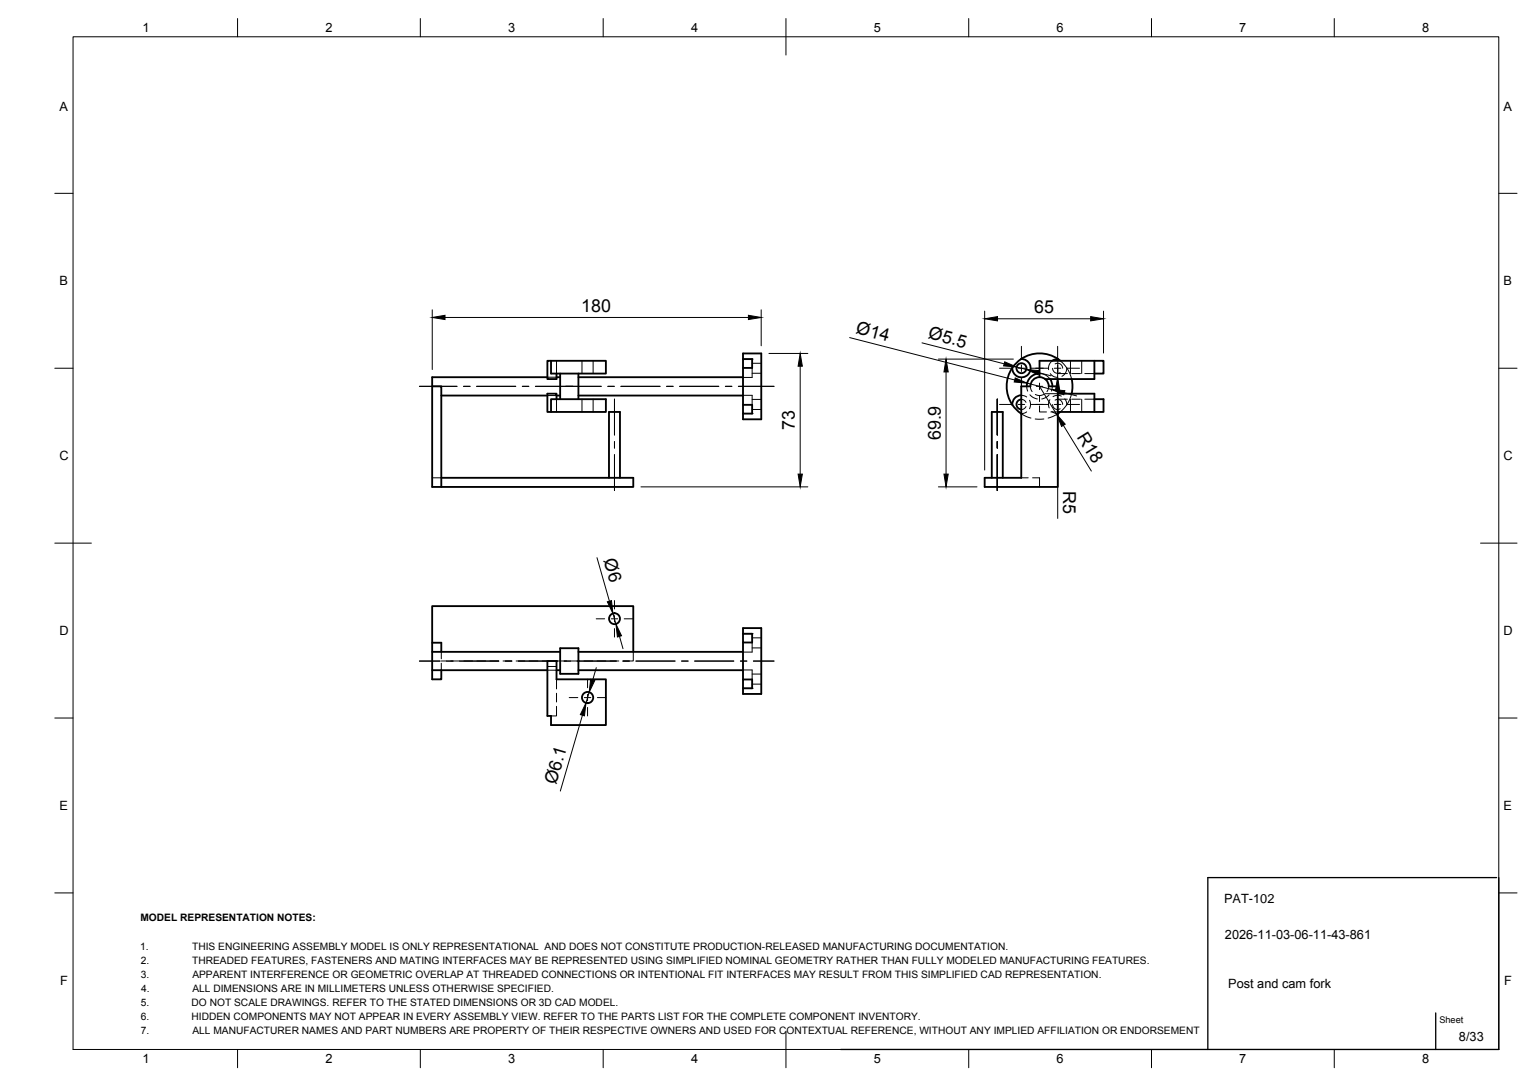
ISO-10303-21;
HEADER;
/* Generated by software containing ST-Developer
 * from STEP Tools, Inc. (www.steptools.com) 
 */

FILE_DESCRIPTION(
/* description */ ('Swing-away clamp arm'),
/* implementation_level */ '2;1');

FILE_NAME(
/* name */ 'Post and cam fork.step',
/* time_stamp */ '2026-10-28T03:26:03-07:00',
/* author */ (''),
/* organization */ (''),
/* preprocessor_version */ 'ST-DEVELOPER v20.2',
/* originating_system */ 'Autodesk Translation Framework v15.17.0.0',
/* authorisation */ '');

FILE_SCHEMA (('AUTOMOTIVE_DESIGN { 1 0 10303 214 3 1 1 }'));
ENDSEC;

DATA;
#10=MECHANICAL_DESIGN_GEOMETRIC_PRESENTATION_REPRESENTATION('',(#296),#10627);
#244=SHAPE_REPRESENTATION_RELATIONSHIP('SRR','None',#10742,#270);
#270=ADVANCED_BREP_SHAPE_REPRESENTATION('',(#330),#10601);
#296=STYLED_ITEM('',(#10958),#330);
#330=MANIFOLD_SOLID_BREP('Body1',#4902);
#366=FACE_BOUND('',#975,.T.);
#367=FACE_BOUND('',#978,.T.);
#368=FACE_BOUND('',#981,.T.);
#369=FACE_BOUND('',#984,.T.);
#370=FACE_BOUND('',#987,.T.);
#371=FACE_BOUND('',#992,.T.);
#372=FACE_BOUND('',#1004,.T.);
#373=FACE_BOUND('',#1005,.T.);
#374=FACE_BOUND('',#1012,.T.);
#375=FACE_BOUND('',#1018,.T.);
#376=FACE_BOUND('',#1022,.T.);
#377=FACE_BOUND('',#1028,.T.);
#378=FACE_BOUND('',#1039,.T.);
#379=FACE_BOUND('',#1042,.T.);
#380=FACE_BOUND('',#1045,.T.);
#381=FACE_BOUND('',#1046,.T.);
#382=FACE_BOUND('',#1047,.T.);
#383=FACE_BOUND('',#1048,.T.);
#476=PLANE('',#5259);
#477=PLANE('',#5265);
#478=PLANE('',#5271);
#479=PLANE('',#5277);
#480=PLANE('',#5283);
#481=PLANE('',#5295);
#482=PLANE('',#5296);
#483=PLANE('',#5297);
#484=PLANE('',#5298);
#485=PLANE('',#5299);
#486=PLANE('',#5300);
#487=PLANE('',#5301);
#488=PLANE('',#5303);
#489=PLANE('',#5304);
#490=PLANE('',#5305);
#491=PLANE('',#5306);
#492=PLANE('',#5307);
#493=PLANE('',#5318);
#494=PLANE('',#5319);
#495=PLANE('',#5320);
#496=PLANE('',#5321);
#497=PLANE('',#5322);
#498=PLANE('',#5323);
#499=PLANE('',#5324);
#500=PLANE('',#5325);
#501=PLANE('',#5326);
#502=PLANE('',#5327);
#503=PLANE('',#5328);
#504=PLANE('',#5332);
#505=PLANE('',#5333);
#506=PLANE('',#5334);
#507=PLANE('',#5335);
#508=PLANE('',#5336);
#509=PLANE('',#5337);
#510=PLANE('',#5338);
#511=PLANE('',#5339);
#512=PLANE('',#5340);
#513=PLANE('',#5341);
#514=PLANE('',#5342);
#515=PLANE('',#5351);
#516=PLANE('',#5356);
#517=PLANE('',#5358);
#659=FACE_OUTER_BOUND('',#974,.T.);
#660=FACE_OUTER_BOUND('',#976,.T.);
#661=FACE_OUTER_BOUND('',#977,.T.);
#662=FACE_OUTER_BOUND('',#979,.T.);
#663=FACE_OUTER_BOUND('',#980,.T.);
#664=FACE_OUTER_BOUND('',#982,.T.);
#665=FACE_OUTER_BOUND('',#983,.T.);
#666=FACE_OUTER_BOUND('',#985,.T.);
#667=FACE_OUTER_BOUND('',#986,.T.);
#668=FACE_OUTER_BOUND('',#988,.T.);
#669=FACE_OUTER_BOUND('',#989,.T.);
#670=FACE_OUTER_BOUND('',#990,.T.);
#671=FACE_OUTER_BOUND('',#991,.T.);
#672=FACE_OUTER_BOUND('',#993,.T.);
#673=FACE_OUTER_BOUND('',#994,.T.);
#674=FACE_OUTER_BOUND('',#995,.T.);
#675=FACE_OUTER_BOUND('',#996,.T.);
#676=FACE_OUTER_BOUND('',#997,.T.);
#677=FACE_OUTER_BOUND('',#998,.T.);
#678=FACE_OUTER_BOUND('',#999,.T.);
#679=FACE_OUTER_BOUND('',#1000,.T.);
#680=FACE_OUTER_BOUND('',#1001,.T.);
#681=FACE_OUTER_BOUND('',#1002,.T.);
#682=FACE_OUTER_BOUND('',#1003,.T.);
#683=FACE_OUTER_BOUND('',#1006,.T.);
#684=FACE_OUTER_BOUND('',#1007,.T.);
#685=FACE_OUTER_BOUND('',#1008,.T.);
#686=FACE_OUTER_BOUND('',#1009,.T.);
#687=FACE_OUTER_BOUND('',#1010,.T.);
#688=FACE_OUTER_BOUND('',#1011,.T.);
#689=FACE_OUTER_BOUND('',#1013,.T.);
#690=FACE_OUTER_BOUND('',#1014,.T.);
#691=FACE_OUTER_BOUND('',#1015,.T.);
#692=FACE_OUTER_BOUND('',#1016,.T.);
#693=FACE_OUTER_BOUND('',#1017,.T.);
#694=FACE_OUTER_BOUND('',#1019,.T.);
#695=FACE_OUTER_BOUND('',#1020,.T.);
#696=FACE_OUTER_BOUND('',#1021,.T.);
#697=FACE_OUTER_BOUND('',#1023,.T.);
#698=FACE_OUTER_BOUND('',#1024,.T.);
#699=FACE_OUTER_BOUND('',#1025,.T.);
#700=FACE_OUTER_BOUND('',#1026,.T.);
#701=FACE_OUTER_BOUND('',#1027,.T.);
#702=FACE_OUTER_BOUND('',#1029,.T.);
#703=FACE_OUTER_BOUND('',#1030,.T.);
#704=FACE_OUTER_BOUND('',#1031,.T.);
#705=FACE_OUTER_BOUND('',#1032,.T.);
#706=FACE_OUTER_BOUND('',#1033,.T.);
#707=FACE_OUTER_BOUND('',#1034,.T.);
#708=FACE_OUTER_BOUND('',#1035,.T.);
#709=FACE_OUTER_BOUND('',#1036,.T.);
#710=FACE_OUTER_BOUND('',#1037,.T.);
#711=FACE_OUTER_BOUND('',#1038,.T.);
#712=FACE_OUTER_BOUND('',#1040,.T.);
#713=FACE_OUTER_BOUND('',#1041,.T.);
#714=FACE_OUTER_BOUND('',#1043,.T.);
#715=FACE_OUTER_BOUND('',#1044,.T.);
#974=EDGE_LOOP('',(#3377,#3378));
#975=EDGE_LOOP('',(#3379));
#976=EDGE_LOOP('',(#3380,#3381,#3382,#3383));
#977=EDGE_LOOP('',(#3384,#3385));
#978=EDGE_LOOP('',(#3386));
#979=EDGE_LOOP('',(#3387,#3388,#3389,#3390));
#980=EDGE_LOOP('',(#3391,#3392));
#981=EDGE_LOOP('',(#3393));
#982=EDGE_LOOP('',(#3394,#3395,#3396,#3397));
#983=EDGE_LOOP('',(#3398,#3399));
#984=EDGE_LOOP('',(#3400));
#985=EDGE_LOOP('',(#3401,#3402,#3403,#3404));
#986=EDGE_LOOP('',(#3405,#3406,#3407,#3408,#3409,#3410,#3411,#3412,#3413));
#987=EDGE_LOOP('',(#3414));
#988=EDGE_LOOP('',(#3415,#3416,#3417,#3418,#3419,#3420,#3421,#3422,#3423,
#3424,#3425,#3426,#3427,#3428,#3429,#3430,#3431,#3432,#3433,#3434));
#989=EDGE_LOOP('',(#3435,#3436,#3437,#3438));
#990=EDGE_LOOP('',(#3439));
#991=EDGE_LOOP('',(#3440,#3441,#3442,#3443,#3444,#3445));
#992=EDGE_LOOP('',(#3446));
#993=EDGE_LOOP('',(#3447,#3448,#3449,#3450));
#994=EDGE_LOOP('',(#3451,#3452,#3453,#3454));
#995=EDGE_LOOP('',(#3455,#3456,#3457,#3458));
#996=EDGE_LOOP('',(#3459,#3460,#3461,#3462));
#997=EDGE_LOOP('',(#3463,#3464,#3465,#3466,#3467,#3468,#3469,#3470));
#998=EDGE_LOOP('',(#3471,#3472,#3473,#3474));
#999=EDGE_LOOP('',(#3475,#3476,#3477,#3478));
#1000=EDGE_LOOP('',(#3479,#3480,#3481,#3482));
#1001=EDGE_LOOP('',(#3483,#3484,#3485,#3486,#3487,#3488));
#1002=EDGE_LOOP('',(#3489,#3490,#3491,#3492,#3493,#3494,#3495,#3496));
#1003=EDGE_LOOP('',(#3497,#3498,#3499,#3500,#3501,#3502,#3503));
#1004=EDGE_LOOP('',(#3504,#3505,#3506,#3507));
#1005=EDGE_LOOP('',(#3508,#3509,#3510,#3511));
#1006=EDGE_LOOP('',(#3512,#3513,#3514,#3515));
#1007=EDGE_LOOP('',(#3516,#3517,#3518,#3519));
#1008=EDGE_LOOP('',(#3520,#3521,#3522,#3523));
#1009=EDGE_LOOP('',(#3524,#3525,#3526,#3527));
#1010=EDGE_LOOP('',(#3528,#3529,#3530,#3531));
#1011=EDGE_LOOP('',(#3532,#3533,#3534,#3535,#3536,#3537));
#1012=EDGE_LOOP('',(#3538));
#1013=EDGE_LOOP('',(#3539,#3540,#3541,#3542,#3543,#3544,#3545));
#1014=EDGE_LOOP('',(#3546,#3547,#3548,#3549,#3550,#3551));
#1015=EDGE_LOOP('',(#3552,#3553,#3554,#3555));
#1016=EDGE_LOOP('',(#3556,#3557,#3558,#3559,#3560));
#1017=EDGE_LOOP('',(#3561,#3562,#3563,#3564,#3565,#3566,#3567,#3568));
#1018=EDGE_LOOP('',(#3569));
#1019=EDGE_LOOP('',(#3570,#3571,#3572,#3573));
#1020=EDGE_LOOP('',(#3574,#3575,#3576,#3577));
#1021=EDGE_LOOP('',(#3578,#3579,#3580,#3581,#3582,#3583));
#1022=EDGE_LOOP('',(#3584));
#1023=EDGE_LOOP('',(#3585,#3586,#3587,#3588));
#1024=EDGE_LOOP('',(#3589,#3590,#3591,#3592));
#1025=EDGE_LOOP('',(#3593,#3594,#3595,#3596));
#1026=EDGE_LOOP('',(#3597,#3598,#3599,#3600));
#1027=EDGE_LOOP('',(#3601,#3602,#3603,#3604,#3605,#3606,#3607,#3608));
#1028=EDGE_LOOP('',(#3609));
#1029=EDGE_LOOP('',(#3610,#3611,#3612,#3613,#3614));
#1030=EDGE_LOOP('',(#3615,#3616,#3617,#3618));
#1031=EDGE_LOOP('',(#3619,#3620,#3621,#3622,#3623,#3624,#3625));
#1032=EDGE_LOOP('',(#3626,#3627,#3628,#3629,#3630,#3631));
#1033=EDGE_LOOP('',(#3632,#3633,#3634,#3635));
#1034=EDGE_LOOP('',(#3636,#3637,#3638,#3639));
#1035=EDGE_LOOP('',(#3640,#3641,#3642,#3643));
#1036=EDGE_LOOP('',(#3644,#3645,#3646,#3647));
#1037=EDGE_LOOP('',(#3648,#3649,#3650,#3651));
#1038=EDGE_LOOP('',(#3652));
#1039=EDGE_LOOP('',(#3653));
#1040=EDGE_LOOP('',(#3654,#3655,#3656,#3657));
#1041=EDGE_LOOP('',(#3658));
#1042=EDGE_LOOP('',(#3659));
#1043=EDGE_LOOP('',(#3660,#3661,#3662,#3663));
#1044=EDGE_LOOP('',(#3664));
#1045=EDGE_LOOP('',(#3665));
#1046=EDGE_LOOP('',(#3666));
#1047=EDGE_LOOP('',(#3667));
#1048=EDGE_LOOP('',(#3668));
#1391=LINE('',#7603,#1713);
#1392=LINE('',#7606,#1714);
#1393=LINE('',#7616,#1715);
#1394=LINE('',#7619,#1716);
#1395=LINE('',#7629,#1717);
#1396=LINE('',#7632,#1718);
#1397=LINE('',#7642,#1719);
#1398=LINE('',#7645,#1720);
#1399=LINE('',#7657,#1721);
#1400=LINE('',#7663,#1722);
#1401=LINE('',#7669,#1723);
#1402=LINE('',#7671,#1724);
#1403=LINE('',#7673,#1725);
#1404=LINE('',#7675,#1726);
#1405=LINE('',#7677,#1727);
#1406=LINE('',#7678,#1728);
#1407=LINE('',#7681,#1729);
#1408=LINE('',#7683,#1730);
#1409=LINE('',#7684,#1731);
#1410=LINE('',#7688,#1732);
#1411=LINE('',#7689,#1733);
#1412=LINE('',#7690,#1734);
#1413=LINE('',#7692,#1735);
#1414=LINE('',#7695,#1736);
#1415=LINE('',#7697,#1737);
#1416=LINE('',#7698,#1738);
#1417=LINE('',#7701,#1739);
#1418=LINE('',#7703,#1740);
#1419=LINE('',#7705,#1741);
#1420=LINE('',#7708,#1742);
#1421=LINE('',#7711,#1743);
#1422=LINE('',#7712,#1744);
#1423=LINE('',#7715,#1745);
#1424=LINE('',#7717,#1746);
#1425=LINE('',#7718,#1747);
#1426=LINE('',#7721,#1748);
#1427=LINE('',#7722,#1749);
#1428=LINE('',#7724,#1750);
#1429=LINE('',#7729,#1751);
#1430=LINE('',#7733,#1752);
#1431=LINE('',#7737,#1753);
#1432=LINE('',#7741,#1754);
#1433=LINE('',#7745,#1755);
#1434=LINE('',#7751,#1756);
#1435=LINE('',#7756,#1757);
#1436=LINE('',#7758,#1758);
#1437=LINE('',#7760,#1759);
#1438=LINE('',#7761,#1760);
#1439=LINE('',#7765,#1761);
#1440=LINE('',#7767,#1762);
#1441=LINE('',#7769,#1763);
#1442=LINE('',#7770,#1764);
#1443=LINE('',#7773,#1765);
#1444=LINE('',#7775,#1766);
#1445=LINE('',#7776,#1767);
#1446=LINE('',#7778,#1768);
#1447=LINE('',#7779,#1769);
#1448=LINE('',#7782,#1770);
#1449=LINE('',#7783,#1771);
#1450=LINE('',#7786,#1772);
#1451=LINE('',#7787,#1773);
#1452=LINE('',#7789,#1774);
#1453=LINE('',#7790,#1775);
#1454=LINE('',#7793,#1776);
#1455=LINE('',#7795,#1777);
#1456=LINE('',#7796,#1778);
#1457=LINE('',#7799,#1779);
#1458=LINE('',#7800,#1780);
#1459=LINE('',#7802,#1781);
#1460=LINE('',#7803,#1782);
#1461=LINE('',#7810,#1783);
#1462=LINE('',#7815,#1784);
#1463=LINE('',#7817,#1785);
#1464=LINE('',#7819,#1786);
#1465=LINE('',#7821,#1787);
#1466=LINE('',#7823,#1788);
#1467=LINE('',#7824,#1789);
#1468=LINE('',#7827,#1790);
#1469=LINE('',#7829,#1791);
#1470=LINE('',#7830,#1792);
#1471=LINE('',#7833,#1793);
#1472=LINE('',#7835,#1794);
#1473=LINE('',#7836,#1795);
#1474=LINE('',#7839,#1796);
#1475=LINE('',#7840,#1797);
#1476=LINE('',#7842,#1798);
#1477=LINE('',#7845,#1799);
#1478=LINE('',#7847,#1800);
#1479=LINE('',#7849,#1801);
#1480=LINE('',#7850,#1802);
#1481=LINE('',#7852,#1803);
#1482=LINE('',#7854,#1804);
#1483=LINE('',#7855,#1805);
#1484=LINE('',#7857,#1806);
#1485=LINE('',#7860,#1807);
#1486=LINE('',#7861,#1808);
#1487=LINE('',#7863,#1809);
#1488=LINE('',#7868,#1810);
#1489=LINE('',#7872,#1811);
#1490=LINE('',#7876,#1812);
#1491=LINE('',#7880,#1813);
#1492=LINE('',#7889,#1814);
#1493=LINE('',#7892,#1815);
#1713=VECTOR('',#5992,1.);
#1714=VECTOR('',#5995,1.);
#1715=VECTOR('',#6006,1.);
#1716=VECTOR('',#6009,1.);
#1717=VECTOR('',#6020,1.);
#1718=VECTOR('',#6023,1.);
#1719=VECTOR('',#6034,1.);
#1720=VECTOR('',#6037,1.);
#1721=VECTOR('',#6054,1.8);
#1722=VECTOR('',#6061,0.3);
#1723=VECTOR('',#6068,1.);
#1724=VECTOR('',#6069,1.);
#1725=VECTOR('',#6070,1.);
#1726=VECTOR('',#6071,1.);
#1727=VECTOR('',#6072,1.);
#1728=VECTOR('',#6073,1.);
#1729=VECTOR('',#6076,1.);
#1730=VECTOR('',#6077,1.);
#1731=VECTOR('',#6078,1.);
#1732=VECTOR('',#6081,1.);
#1733=VECTOR('',#6082,1.);
#1734=VECTOR('',#6083,1.);
#1735=VECTOR('',#6086,1.);
#1736=VECTOR('',#6089,1.);
#1737=VECTOR('',#6090,1.);
#1738=VECTOR('',#6091,1.);
#1739=VECTOR('',#6094,1.);
#1740=VECTOR('',#6095,1.);
#1741=VECTOR('',#6096,1.);
#1742=VECTOR('',#6099,1.);
#1743=VECTOR('',#6102,1.);
#1744=VECTOR('',#6103,1.);
#1745=VECTOR('',#6106,1.);
#1746=VECTOR('',#6107,1.);
#1747=VECTOR('',#6108,1.);
#1748=VECTOR('',#6111,1.);
#1749=VECTOR('',#6112,1.);
#1750=VECTOR('',#6115,1.);
#1751=VECTOR('',#6122,0.5);
#1752=VECTOR('',#6125,1.);
#1753=VECTOR('',#6128,1.);
#1754=VECTOR('',#6131,1.);
#1755=VECTOR('',#6134,1.);
#1756=VECTOR('',#6141,0.305);
#1757=VECTOR('',#6146,1.);
#1758=VECTOR('',#6147,1.);
#1759=VECTOR('',#6148,1.);
#1760=VECTOR('',#6149,1.);
#1761=VECTOR('',#6152,1.);
#1762=VECTOR('',#6153,1.);
#1763=VECTOR('',#6154,1.);
#1764=VECTOR('',#6155,1.);
#1765=VECTOR('',#6158,1.);
#1766=VECTOR('',#6159,1.);
#1767=VECTOR('',#6160,1.);
#1768=VECTOR('',#6163,1.);
#1769=VECTOR('',#6164,1.);
#1770=VECTOR('',#6167,1.);
#1771=VECTOR('',#6168,1.);
#1772=VECTOR('',#6171,1.);
#1773=VECTOR('',#6172,1.);
#1774=VECTOR('',#6173,1.);
#1775=VECTOR('',#6174,1.);
#1776=VECTOR('',#6177,1.);
#1777=VECTOR('',#6178,1.);
#1778=VECTOR('',#6179,1.);
#1779=VECTOR('',#6182,1.);
#1780=VECTOR('',#6183,1.);
#1781=VECTOR('',#6186,1.);
#1782=VECTOR('',#6187,1.);
#1783=VECTOR('',#6196,0.305);
#1784=VECTOR('',#6201,1.);
#1785=VECTOR('',#6202,1.);
#1786=VECTOR('',#6203,1.);
#1787=VECTOR('',#6204,1.);
#1788=VECTOR('',#6205,1.);
#1789=VECTOR('',#6206,1.);
#1790=VECTOR('',#6209,1.);
#1791=VECTOR('',#6210,1.);
#1792=VECTOR('',#6211,1.);
#1793=VECTOR('',#6214,1.);
#1794=VECTOR('',#6215,1.);
#1795=VECTOR('',#6216,1.);
#1796=VECTOR('',#6219,1.);
#1797=VECTOR('',#6220,1.);
#1798=VECTOR('',#6223,1.);
#1799=VECTOR('',#6226,1.);
#1800=VECTOR('',#6227,1.);
#1801=VECTOR('',#6228,1.);
#1802=VECTOR('',#6229,1.);
#1803=VECTOR('',#6232,1.);
#1804=VECTOR('',#6233,1.);
#1805=VECTOR('',#6234,1.);
#1806=VECTOR('',#6237,1.);
#1807=VECTOR('',#6240,1.);
#1808=VECTOR('',#6241,1.);
#1809=VECTOR('',#6244,1.);
#1810=VECTOR('',#6251,0.275);
#1811=VECTOR('',#6256,0.275);
#1812=VECTOR('',#6261,0.275);
#1813=VECTOR('',#6266,0.275);
#1814=VECTOR('',#6277,0.7);
#1815=VECTOR('',#6282,0.5);
#2003=CIRCLE('',#5260,1.8);
#2004=CIRCLE('',#5261,0.5);
#2005=CIRCLE('',#5262,0.275);
#2006=CIRCLE('',#5264,0.5);
#2007=CIRCLE('',#5266,1.8);
#2008=CIRCLE('',#5267,0.5);
#2009=CIRCLE('',#5268,0.275);
#2010=CIRCLE('',#5270,0.5);
#2011=CIRCLE('',#5272,1.8);
#2012=CIRCLE('',#5273,0.5);
#2013=CIRCLE('',#5274,0.275);
#2014=CIRCLE('',#5276,0.5);
#2015=CIRCLE('',#5278,1.8);
#2016=CIRCLE('',#5279,0.5);
#2017=CIRCLE('',#5280,0.275);
#2018=CIRCLE('',#5282,0.5);
#2019=CIRCLE('',#5284,1.8);
#2020=CIRCLE('',#5285,1.8);
#2021=CIRCLE('',#5286,1.8);
#2022=CIRCLE('',#5287,1.8);
#2023=CIRCLE('',#5288,1.8);
#2024=CIRCLE('',#5289,0.5);
#2025=CIRCLE('',#5291,1.8);
#2026=CIRCLE('',#5293,0.3);
#2027=CIRCLE('',#5294,0.3);
#2028=CIRCLE('',#5302,0.5);
#2029=CIRCLE('',#5308,0.5);
#2030=CIRCLE('',#5310,0.5);
#2031=CIRCLE('',#5311,0.5);
#2032=CIRCLE('',#5312,0.5);
#2033=CIRCLE('',#5313,0.5);
#2034=CIRCLE('',#5314,0.5);
#2035=CIRCLE('',#5316,0.305);
#2036=CIRCLE('',#5317,0.305);
#2037=CIRCLE('',#5330,0.305);
#2038=CIRCLE('',#5331,0.305);
#2039=CIRCLE('',#5344,0.275);
#2040=CIRCLE('',#5346,0.275);
#2041=CIRCLE('',#5348,0.275);
#2042=CIRCLE('',#5350,0.275);
#2043=CIRCLE('',#5352,0.7);
#2044=CIRCLE('',#5353,0.5);
#2045=CIRCLE('',#5355,0.7);
#2294=VERTEX_POINT('',#7595);
#2295=VERTEX_POINT('',#7596);
#2296=VERTEX_POINT('',#7599);
#2297=VERTEX_POINT('',#7602);
#2298=VERTEX_POINT('',#7604);
#2299=VERTEX_POINT('',#7608);
#2300=VERTEX_POINT('',#7609);
#2301=VERTEX_POINT('',#7612);
#2302=VERTEX_POINT('',#7615);
#2303=VERTEX_POINT('',#7617);
#2304=VERTEX_POINT('',#7621);
#2305=VERTEX_POINT('',#7622);
#2306=VERTEX_POINT('',#7625);
#2307=VERTEX_POINT('',#7628);
#2308=VERTEX_POINT('',#7630);
#2309=VERTEX_POINT('',#7634);
#2310=VERTEX_POINT('',#7635);
#2311=VERTEX_POINT('',#7638);
#2312=VERTEX_POINT('',#7641);
#2313=VERTEX_POINT('',#7643);
#2314=VERTEX_POINT('',#7650);
#2315=VERTEX_POINT('',#7653);
#2316=VERTEX_POINT('',#7656);
#2317=VERTEX_POINT('',#7660);
#2318=VERTEX_POINT('',#7662);
#2319=VERTEX_POINT('',#7667);
#2320=VERTEX_POINT('',#7668);
#2321=VERTEX_POINT('',#7670);
#2322=VERTEX_POINT('',#7672);
#2323=VERTEX_POINT('',#7674);
#2324=VERTEX_POINT('',#7676);
#2325=VERTEX_POINT('',#7680);
#2326=VERTEX_POINT('',#7682);
#2327=VERTEX_POINT('',#7686);
#2328=VERTEX_POINT('',#7687);
#2329=VERTEX_POINT('',#7694);
#2330=VERTEX_POINT('',#7696);
#2331=VERTEX_POINT('',#7700);
#2332=VERTEX_POINT('',#7702);
#2333=VERTEX_POINT('',#7704);
#2334=VERTEX_POINT('',#7706);
#2335=VERTEX_POINT('',#7710);
#2336=VERTEX_POINT('',#7714);
#2337=VERTEX_POINT('',#7716);
#2338=VERTEX_POINT('',#7720);
#2339=VERTEX_POINT('',#7728);
#2340=VERTEX_POINT('',#7731);
#2341=VERTEX_POINT('',#7732);
#2342=VERTEX_POINT('',#7734);
#2343=VERTEX_POINT('',#7736);
#2344=VERTEX_POINT('',#7739);
#2345=VERTEX_POINT('',#7740);
#2346=VERTEX_POINT('',#7742);
#2347=VERTEX_POINT('',#7744);
#2348=VERTEX_POINT('',#7748);
#2349=VERTEX_POINT('',#7750);
#2350=VERTEX_POINT('',#7754);
#2351=VERTEX_POINT('',#7755);
#2352=VERTEX_POINT('',#7757);
#2353=VERTEX_POINT('',#7759);
#2354=VERTEX_POINT('',#7763);
#2355=VERTEX_POINT('',#7764);
#2356=VERTEX_POINT('',#7766);
#2357=VERTEX_POINT('',#7768);
#2358=VERTEX_POINT('',#7772);
#2359=VERTEX_POINT('',#7774);
#2360=VERTEX_POINT('',#7781);
#2361=VERTEX_POINT('',#7785);
#2362=VERTEX_POINT('',#7788);
#2363=VERTEX_POINT('',#7792);
#2364=VERTEX_POINT('',#7794);
#2365=VERTEX_POINT('',#7798);
#2366=VERTEX_POINT('',#7807);
#2367=VERTEX_POINT('',#7809);
#2368=VERTEX_POINT('',#7813);
#2369=VERTEX_POINT('',#7814);
#2370=VERTEX_POINT('',#7816);
#2371=VERTEX_POINT('',#7818);
#2372=VERTEX_POINT('',#7820);
#2373=VERTEX_POINT('',#7822);
#2374=VERTEX_POINT('',#7826);
#2375=VERTEX_POINT('',#7828);
#2376=VERTEX_POINT('',#7832);
#2377=VERTEX_POINT('',#7834);
#2378=VERTEX_POINT('',#7838);
#2379=VERTEX_POINT('',#7844);
#2380=VERTEX_POINT('',#7846);
#2381=VERTEX_POINT('',#7848);
#2382=VERTEX_POINT('',#7853);
#2383=VERTEX_POINT('',#7859);
#2384=VERTEX_POINT('',#7866);
#2385=VERTEX_POINT('',#7870);
#2386=VERTEX_POINT('',#7874);
#2387=VERTEX_POINT('',#7878);
#2388=VERTEX_POINT('',#7882);
#2389=VERTEX_POINT('',#7884);
#2390=VERTEX_POINT('',#7887);
#2721=EDGE_CURVE('',#2294,#2295,#2003,.T.);
#2722=EDGE_CURVE('',#2294,#2295,#2004,.T.);
#2723=EDGE_CURVE('',#2296,#2296,#2005,.T.);
#2724=EDGE_CURVE('',#2297,#2294,#1391,.T.);
#2725=EDGE_CURVE('',#2298,#2297,#2006,.T.);
#2726=EDGE_CURVE('',#2295,#2298,#1392,.T.);
#2727=EDGE_CURVE('',#2299,#2300,#2007,.T.);
#2728=EDGE_CURVE('',#2299,#2300,#2008,.T.);
#2729=EDGE_CURVE('',#2301,#2301,#2009,.T.);
#2730=EDGE_CURVE('',#2302,#2299,#1393,.T.);
#2731=EDGE_CURVE('',#2303,#2302,#2010,.T.);
#2732=EDGE_CURVE('',#2300,#2303,#1394,.T.);
#2733=EDGE_CURVE('',#2304,#2305,#2011,.T.);
#2734=EDGE_CURVE('',#2304,#2305,#2012,.T.);
#2735=EDGE_CURVE('',#2306,#2306,#2013,.T.);
#2736=EDGE_CURVE('',#2307,#2304,#1395,.T.);
#2737=EDGE_CURVE('',#2308,#2307,#2014,.T.);
#2738=EDGE_CURVE('',#2305,#2308,#1396,.T.);
#2739=EDGE_CURVE('',#2309,#2310,#2015,.T.);
#2740=EDGE_CURVE('',#2309,#2310,#2016,.T.);
#2741=EDGE_CURVE('',#2311,#2311,#2017,.T.);
#2742=EDGE_CURVE('',#2312,#2309,#1397,.T.);
#2743=EDGE_CURVE('',#2313,#2312,#2018,.T.);
#2744=EDGE_CURVE('',#2310,#2313,#1398,.T.);
#2745=EDGE_CURVE('',#2297,#2313,#2019,.T.);
#2746=EDGE_CURVE('',#2312,#2308,#2020,.T.);
#2747=EDGE_CURVE('',#2307,#2303,#2021,.T.);
#2748=EDGE_CURVE('',#2302,#2314,#2022,.T.);
#2749=EDGE_CURVE('',#2314,#2298,#2023,.T.);
#2750=EDGE_CURVE('',#2315,#2315,#2024,.T.);
#2751=EDGE_CURVE('',#2314,#2316,#1399,.T.);
#2752=EDGE_CURVE('',#2316,#2316,#2025,.T.);
#2753=EDGE_CURVE('',#2317,#2317,#2026,.T.);
#2754=EDGE_CURVE('',#2317,#2318,#1400,.T.);
#2755=EDGE_CURVE('',#2318,#2318,#2027,.T.);
#2756=EDGE_CURVE('',#2319,#2320,#1401,.T.);
#2757=EDGE_CURVE('',#2321,#2319,#1402,.T.);
#2758=EDGE_CURVE('',#2321,#2322,#1403,.T.);
#2759=EDGE_CURVE('',#2322,#2323,#1404,.T.);
#2760=EDGE_CURVE('',#2323,#2324,#1405,.T.);
#2761=EDGE_CURVE('',#2324,#2320,#1406,.T.);
#2762=EDGE_CURVE('',#2325,#2321,#1407,.T.);
#2763=EDGE_CURVE('',#2326,#2325,#1408,.T.);
#2764=EDGE_CURVE('',#2326,#2322,#1409,.T.);
#2765=EDGE_CURVE('',#2327,#2328,#1410,.T.);
#2766=EDGE_CURVE('',#2327,#2324,#1411,.T.);
#2767=EDGE_CURVE('',#2328,#2323,#1412,.T.);
#2768=EDGE_CURVE('',#2328,#2326,#1413,.T.);
#2769=EDGE_CURVE('',#2329,#2320,#1414,.T.);
#2770=EDGE_CURVE('',#2330,#2329,#1415,.T.);
#2771=EDGE_CURVE('',#2330,#2319,#1416,.T.);
#2772=EDGE_CURVE('',#2331,#2327,#1417,.T.);
#2773=EDGE_CURVE('',#2331,#2332,#1418,.T.);
#2774=EDGE_CURVE('',#2332,#2333,#1419,.T.);
#2775=EDGE_CURVE('',#2333,#2334,#2028,.T.);
#2776=EDGE_CURVE('',#2334,#2329,#1420,.T.);
#2777=EDGE_CURVE('',#2335,#2334,#1421,.T.);
#2778=EDGE_CURVE('',#2335,#2330,#1422,.T.);
#2779=EDGE_CURVE('',#2333,#2336,#1423,.T.);
#2780=EDGE_CURVE('',#2337,#2332,#1424,.T.);
#2781=EDGE_CURVE('',#2337,#2336,#1425,.T.);
#2782=EDGE_CURVE('',#2338,#2337,#1426,.T.);
#2783=EDGE_CURVE('',#2338,#2331,#1427,.T.);
#2784=EDGE_CURVE('',#2325,#2338,#1428,.T.);
#2785=EDGE_CURVE('',#2336,#2335,#2029,.T.);
#2786=EDGE_CURVE('',#2335,#2339,#1429,.T.);
#2787=EDGE_CURVE('',#2339,#2339,#2030,.T.);
#2788=EDGE_CURVE('',#2340,#2341,#1430,.T.);
#2789=EDGE_CURVE('',#2341,#2342,#2031,.T.);
#2790=EDGE_CURVE('',#2342,#2343,#1431,.T.);
#2791=EDGE_CURVE('',#2343,#2340,#2032,.T.);
#2792=EDGE_CURVE('',#2344,#2345,#1432,.T.);
#2793=EDGE_CURVE('',#2345,#2346,#2033,.T.);
#2794=EDGE_CURVE('',#2346,#2347,#1433,.T.);
#2795=EDGE_CURVE('',#2347,#2344,#2034,.T.);
#2796=EDGE_CURVE('',#2348,#2348,#2035,.T.);
#2797=EDGE_CURVE('',#2348,#2349,#1434,.T.);
#2798=EDGE_CURVE('',#2349,#2349,#2036,.T.);
#2799=EDGE_CURVE('',#2350,#2351,#1435,.T.);
#2800=EDGE_CURVE('',#2352,#2350,#1436,.T.);
#2801=EDGE_CURVE('',#2352,#2353,#1437,.T.);
#2802=EDGE_CURVE('',#2351,#2353,#1438,.T.);
#2803=EDGE_CURVE('',#2354,#2355,#1439,.T.);
#2804=EDGE_CURVE('',#2356,#2354,#1440,.T.);
#2805=EDGE_CURVE('',#2357,#2356,#1441,.T.);
#2806=EDGE_CURVE('',#2355,#2357,#1442,.T.);
#2807=EDGE_CURVE('',#2357,#2358,#1443,.T.);
#2808=EDGE_CURVE('',#2359,#2356,#1444,.T.);
#2809=EDGE_CURVE('',#2358,#2359,#1445,.T.);
#2810=EDGE_CURVE('',#2358,#2352,#1446,.T.);
#2811=EDGE_CURVE('',#2353,#2359,#1447,.T.);
#2812=EDGE_CURVE('',#2355,#2360,#1448,.T.);
#2813=EDGE_CURVE('',#2360,#2350,#1449,.T.);
#2814=EDGE_CURVE('',#2361,#2360,#1450,.T.);
#2815=EDGE_CURVE('',#2346,#2361,#1451,.T.);
#2816=EDGE_CURVE('',#2345,#2362,#1452,.T.);
#2817=EDGE_CURVE('',#2354,#2362,#1453,.T.);
#2818=EDGE_CURVE('',#2363,#2351,#1454,.T.);
#2819=EDGE_CURVE('',#2364,#2363,#1455,.T.);
#2820=EDGE_CURVE('',#2361,#2364,#1456,.T.);
#2821=EDGE_CURVE('',#2344,#2365,#1457,.T.);
#2822=EDGE_CURVE('',#2362,#2365,#1458,.T.);
#2823=EDGE_CURVE('',#2364,#2347,#1459,.T.);
#2824=EDGE_CURVE('',#2365,#2363,#1460,.T.);
#2825=EDGE_CURVE('',#2366,#2366,#2037,.T.);
#2826=EDGE_CURVE('',#2366,#2367,#1461,.T.);
#2827=EDGE_CURVE('',#2367,#2367,#2038,.T.);
#2828=EDGE_CURVE('',#2368,#2369,#1462,.T.);
#2829=EDGE_CURVE('',#2370,#2368,#1463,.T.);
#2830=EDGE_CURVE('',#2370,#2371,#1464,.T.);
#2831=EDGE_CURVE('',#2371,#2372,#1465,.T.);
#2832=EDGE_CURVE('',#2372,#2373,#1466,.T.);
#2833=EDGE_CURVE('',#2373,#2369,#1467,.T.);
#2834=EDGE_CURVE('',#2374,#2370,#1468,.T.);
#2835=EDGE_CURVE('',#2375,#2374,#1469,.T.);
#2836=EDGE_CURVE('',#2375,#2371,#1470,.T.);
#2837=EDGE_CURVE('',#2369,#2376,#1471,.T.);
#2838=EDGE_CURVE('',#2377,#2373,#1472,.T.);
#2839=EDGE_CURVE('',#2376,#2377,#1473,.T.);
#2840=EDGE_CURVE('',#2377,#2378,#1474,.T.);
#2841=EDGE_CURVE('',#2378,#2372,#1475,.T.);
#2842=EDGE_CURVE('',#2378,#2375,#1476,.T.);
#2843=EDGE_CURVE('',#2374,#2379,#1477,.T.);
#2844=EDGE_CURVE('',#2379,#2380,#1478,.T.);
#2845=EDGE_CURVE('',#2380,#2381,#1479,.T.);
#2846=EDGE_CURVE('',#2381,#2376,#1480,.T.);
#2847=EDGE_CURVE('',#2380,#2341,#1481,.T.);
#2848=EDGE_CURVE('',#2379,#2382,#1482,.T.);
#2849=EDGE_CURVE('',#2342,#2382,#1483,.T.);
#2850=EDGE_CURVE('',#2381,#2340,#1484,.T.);
#2851=EDGE_CURVE('',#2383,#2343,#1485,.T.);
#2852=EDGE_CURVE('',#2368,#2383,#1486,.T.);
#2853=EDGE_CURVE('',#2382,#2383,#1487,.T.);
#2854=EDGE_CURVE('',#2384,#2384,#2039,.T.);
#2855=EDGE_CURVE('',#2384,#2296,#1488,.T.);
#2856=EDGE_CURVE('',#2385,#2385,#2040,.T.);
#2857=EDGE_CURVE('',#2385,#2301,#1489,.T.);
#2858=EDGE_CURVE('',#2386,#2386,#2041,.T.);
#2859=EDGE_CURVE('',#2386,#2306,#1490,.T.);
#2860=EDGE_CURVE('',#2387,#2387,#2042,.T.);
#2861=EDGE_CURVE('',#2387,#2311,#1491,.T.);
#2862=EDGE_CURVE('',#2388,#2388,#2043,.T.);
#2863=EDGE_CURVE('',#2389,#2389,#2044,.T.);
#2864=EDGE_CURVE('',#2390,#2390,#2045,.T.);
#2865=EDGE_CURVE('',#2390,#2388,#1492,.T.);
#2866=EDGE_CURVE('',#2389,#2315,#1493,.T.);
#3377=ORIENTED_EDGE('',*,*,#2721,.F.);
#3378=ORIENTED_EDGE('',*,*,#2722,.T.);
#3379=ORIENTED_EDGE('',*,*,#2723,.F.);
#3380=ORIENTED_EDGE('',*,*,#2724,.F.);
#3381=ORIENTED_EDGE('',*,*,#2725,.F.);
#3382=ORIENTED_EDGE('',*,*,#2726,.F.);
#3383=ORIENTED_EDGE('',*,*,#2722,.F.);
#3384=ORIENTED_EDGE('',*,*,#2727,.F.);
#3385=ORIENTED_EDGE('',*,*,#2728,.T.);
#3386=ORIENTED_EDGE('',*,*,#2729,.F.);
#3387=ORIENTED_EDGE('',*,*,#2730,.F.);
#3388=ORIENTED_EDGE('',*,*,#2731,.F.);
#3389=ORIENTED_EDGE('',*,*,#2732,.F.);
#3390=ORIENTED_EDGE('',*,*,#2728,.F.);
#3391=ORIENTED_EDGE('',*,*,#2733,.F.);
#3392=ORIENTED_EDGE('',*,*,#2734,.T.);
#3393=ORIENTED_EDGE('',*,*,#2735,.F.);
#3394=ORIENTED_EDGE('',*,*,#2736,.F.);
#3395=ORIENTED_EDGE('',*,*,#2737,.F.);
#3396=ORIENTED_EDGE('',*,*,#2738,.F.);
#3397=ORIENTED_EDGE('',*,*,#2734,.F.);
#3398=ORIENTED_EDGE('',*,*,#2739,.F.);
#3399=ORIENTED_EDGE('',*,*,#2740,.T.);
#3400=ORIENTED_EDGE('',*,*,#2741,.F.);
#3401=ORIENTED_EDGE('',*,*,#2742,.F.);
#3402=ORIENTED_EDGE('',*,*,#2743,.F.);
#3403=ORIENTED_EDGE('',*,*,#2744,.F.);
#3404=ORIENTED_EDGE('',*,*,#2740,.F.);
#3405=ORIENTED_EDGE('',*,*,#2725,.T.);
#3406=ORIENTED_EDGE('',*,*,#2745,.T.);
#3407=ORIENTED_EDGE('',*,*,#2743,.T.);
#3408=ORIENTED_EDGE('',*,*,#2746,.T.);
#3409=ORIENTED_EDGE('',*,*,#2737,.T.);
#3410=ORIENTED_EDGE('',*,*,#2747,.T.);
#3411=ORIENTED_EDGE('',*,*,#2731,.T.);
#3412=ORIENTED_EDGE('',*,*,#2748,.T.);
#3413=ORIENTED_EDGE('',*,*,#2749,.T.);
#3414=ORIENTED_EDGE('',*,*,#2750,.T.);
#3415=ORIENTED_EDGE('',*,*,#2724,.T.);
#3416=ORIENTED_EDGE('',*,*,#2721,.T.);
#3417=ORIENTED_EDGE('',*,*,#2726,.T.);
#3418=ORIENTED_EDGE('',*,*,#2749,.F.);
#3419=ORIENTED_EDGE('',*,*,#2751,.T.);
#3420=ORIENTED_EDGE('',*,*,#2752,.T.);
#3421=ORIENTED_EDGE('',*,*,#2751,.F.);
#3422=ORIENTED_EDGE('',*,*,#2748,.F.);
#3423=ORIENTED_EDGE('',*,*,#2730,.T.);
#3424=ORIENTED_EDGE('',*,*,#2727,.T.);
#3425=ORIENTED_EDGE('',*,*,#2732,.T.);
#3426=ORIENTED_EDGE('',*,*,#2747,.F.);
#3427=ORIENTED_EDGE('',*,*,#2736,.T.);
#3428=ORIENTED_EDGE('',*,*,#2733,.T.);
#3429=ORIENTED_EDGE('',*,*,#2738,.T.);
#3430=ORIENTED_EDGE('',*,*,#2746,.F.);
#3431=ORIENTED_EDGE('',*,*,#2742,.T.);
#3432=ORIENTED_EDGE('',*,*,#2739,.T.);
#3433=ORIENTED_EDGE('',*,*,#2744,.T.);
#3434=ORIENTED_EDGE('',*,*,#2745,.F.);
#3435=ORIENTED_EDGE('',*,*,#2753,.F.);
#3436=ORIENTED_EDGE('',*,*,#2754,.T.);
#3437=ORIENTED_EDGE('',*,*,#2755,.F.);
#3438=ORIENTED_EDGE('',*,*,#2754,.F.);
#3439=ORIENTED_EDGE('',*,*,#2753,.T.);
#3440=ORIENTED_EDGE('',*,*,#2756,.F.);
#3441=ORIENTED_EDGE('',*,*,#2757,.F.);
#3442=ORIENTED_EDGE('',*,*,#2758,.T.);
#3443=ORIENTED_EDGE('',*,*,#2759,.T.);
#3444=ORIENTED_EDGE('',*,*,#2760,.T.);
#3445=ORIENTED_EDGE('',*,*,#2761,.T.);
#3446=ORIENTED_EDGE('',*,*,#2755,.T.);
#3447=ORIENTED_EDGE('',*,*,#2762,.F.);
#3448=ORIENTED_EDGE('',*,*,#2763,.F.);
#3449=ORIENTED_EDGE('',*,*,#2764,.T.);
#3450=ORIENTED_EDGE('',*,*,#2758,.F.);
#3451=ORIENTED_EDGE('',*,*,#2765,.F.);
#3452=ORIENTED_EDGE('',*,*,#2766,.T.);
#3453=ORIENTED_EDGE('',*,*,#2760,.F.);
#3454=ORIENTED_EDGE('',*,*,#2767,.F.);
#3455=ORIENTED_EDGE('',*,*,#2768,.F.);
#3456=ORIENTED_EDGE('',*,*,#2767,.T.);
#3457=ORIENTED_EDGE('',*,*,#2759,.F.);
#3458=ORIENTED_EDGE('',*,*,#2764,.F.);
#3459=ORIENTED_EDGE('',*,*,#2756,.T.);
#3460=ORIENTED_EDGE('',*,*,#2769,.F.);
#3461=ORIENTED_EDGE('',*,*,#2770,.F.);
#3462=ORIENTED_EDGE('',*,*,#2771,.T.);
#3463=ORIENTED_EDGE('',*,*,#2772,.F.);
#3464=ORIENTED_EDGE('',*,*,#2773,.T.);
#3465=ORIENTED_EDGE('',*,*,#2774,.T.);
#3466=ORIENTED_EDGE('',*,*,#2775,.T.);
#3467=ORIENTED_EDGE('',*,*,#2776,.T.);
#3468=ORIENTED_EDGE('',*,*,#2769,.T.);
#3469=ORIENTED_EDGE('',*,*,#2761,.F.);
#3470=ORIENTED_EDGE('',*,*,#2766,.F.);
#3471=ORIENTED_EDGE('',*,*,#2777,.F.);
#3472=ORIENTED_EDGE('',*,*,#2778,.T.);
#3473=ORIENTED_EDGE('',*,*,#2770,.T.);
#3474=ORIENTED_EDGE('',*,*,#2776,.F.);
#3475=ORIENTED_EDGE('',*,*,#2779,.F.);
#3476=ORIENTED_EDGE('',*,*,#2774,.F.);
#3477=ORIENTED_EDGE('',*,*,#2780,.F.);
#3478=ORIENTED_EDGE('',*,*,#2781,.T.);
#3479=ORIENTED_EDGE('',*,*,#2782,.T.);
#3480=ORIENTED_EDGE('',*,*,#2780,.T.);
#3481=ORIENTED_EDGE('',*,*,#2773,.F.);
#3482=ORIENTED_EDGE('',*,*,#2783,.F.);
#3483=ORIENTED_EDGE('',*,*,#2784,.T.);
#3484=ORIENTED_EDGE('',*,*,#2783,.T.);
#3485=ORIENTED_EDGE('',*,*,#2772,.T.);
#3486=ORIENTED_EDGE('',*,*,#2765,.T.);
#3487=ORIENTED_EDGE('',*,*,#2768,.T.);
#3488=ORIENTED_EDGE('',*,*,#2763,.T.);
#3489=ORIENTED_EDGE('',*,*,#2757,.T.);
#3490=ORIENTED_EDGE('',*,*,#2771,.F.);
#3491=ORIENTED_EDGE('',*,*,#2778,.F.);
#3492=ORIENTED_EDGE('',*,*,#2785,.F.);
#3493=ORIENTED_EDGE('',*,*,#2781,.F.);
#3494=ORIENTED_EDGE('',*,*,#2782,.F.);
#3495=ORIENTED_EDGE('',*,*,#2784,.F.);
#3496=ORIENTED_EDGE('',*,*,#2762,.T.);
#3497=ORIENTED_EDGE('',*,*,#2779,.T.);
#3498=ORIENTED_EDGE('',*,*,#2785,.T.);
#3499=ORIENTED_EDGE('',*,*,#2786,.T.);
#3500=ORIENTED_EDGE('',*,*,#2787,.F.);
#3501=ORIENTED_EDGE('',*,*,#2786,.F.);
#3502=ORIENTED_EDGE('',*,*,#2777,.T.);
#3503=ORIENTED_EDGE('',*,*,#2775,.F.);
#3504=ORIENTED_EDGE('',*,*,#2788,.T.);
#3505=ORIENTED_EDGE('',*,*,#2789,.T.);
#3506=ORIENTED_EDGE('',*,*,#2790,.T.);
#3507=ORIENTED_EDGE('',*,*,#2791,.T.);
#3508=ORIENTED_EDGE('',*,*,#2792,.T.);
#3509=ORIENTED_EDGE('',*,*,#2793,.T.);
#3510=ORIENTED_EDGE('',*,*,#2794,.T.);
#3511=ORIENTED_EDGE('',*,*,#2795,.T.);
#3512=ORIENTED_EDGE('',*,*,#2796,.F.);
#3513=ORIENTED_EDGE('',*,*,#2797,.T.);
#3514=ORIENTED_EDGE('',*,*,#2798,.F.);
#3515=ORIENTED_EDGE('',*,*,#2797,.F.);
#3516=ORIENTED_EDGE('',*,*,#2799,.F.);
#3517=ORIENTED_EDGE('',*,*,#2800,.F.);
#3518=ORIENTED_EDGE('',*,*,#2801,.T.);
#3519=ORIENTED_EDGE('',*,*,#2802,.F.);
#3520=ORIENTED_EDGE('',*,*,#2803,.F.);
#3521=ORIENTED_EDGE('',*,*,#2804,.F.);
#3522=ORIENTED_EDGE('',*,*,#2805,.F.);
#3523=ORIENTED_EDGE('',*,*,#2806,.F.);
#3524=ORIENTED_EDGE('',*,*,#2807,.F.);
#3525=ORIENTED_EDGE('',*,*,#2805,.T.);
#3526=ORIENTED_EDGE('',*,*,#2808,.F.);
#3527=ORIENTED_EDGE('',*,*,#2809,.F.);
#3528=ORIENTED_EDGE('',*,*,#2810,.F.);
#3529=ORIENTED_EDGE('',*,*,#2809,.T.);
#3530=ORIENTED_EDGE('',*,*,#2811,.F.);
#3531=ORIENTED_EDGE('',*,*,#2801,.F.);
#3532=ORIENTED_EDGE('',*,*,#2812,.F.);
#3533=ORIENTED_EDGE('',*,*,#2806,.T.);
#3534=ORIENTED_EDGE('',*,*,#2807,.T.);
#3535=ORIENTED_EDGE('',*,*,#2810,.T.);
#3536=ORIENTED_EDGE('',*,*,#2800,.T.);
#3537=ORIENTED_EDGE('',*,*,#2813,.F.);
#3538=ORIENTED_EDGE('',*,*,#2796,.T.);
#3539=ORIENTED_EDGE('',*,*,#2803,.T.);
#3540=ORIENTED_EDGE('',*,*,#2812,.T.);
#3541=ORIENTED_EDGE('',*,*,#2814,.F.);
#3542=ORIENTED_EDGE('',*,*,#2815,.F.);
#3543=ORIENTED_EDGE('',*,*,#2793,.F.);
#3544=ORIENTED_EDGE('',*,*,#2816,.T.);
#3545=ORIENTED_EDGE('',*,*,#2817,.F.);
#3546=ORIENTED_EDGE('',*,*,#2813,.T.);
#3547=ORIENTED_EDGE('',*,*,#2799,.T.);
#3548=ORIENTED_EDGE('',*,*,#2818,.F.);
#3549=ORIENTED_EDGE('',*,*,#2819,.F.);
#3550=ORIENTED_EDGE('',*,*,#2820,.F.);
#3551=ORIENTED_EDGE('',*,*,#2814,.T.);
#3552=ORIENTED_EDGE('',*,*,#2792,.F.);
#3553=ORIENTED_EDGE('',*,*,#2821,.T.);
#3554=ORIENTED_EDGE('',*,*,#2822,.F.);
#3555=ORIENTED_EDGE('',*,*,#2816,.F.);
#3556=ORIENTED_EDGE('',*,*,#2795,.F.);
#3557=ORIENTED_EDGE('',*,*,#2823,.F.);
#3558=ORIENTED_EDGE('',*,*,#2819,.T.);
#3559=ORIENTED_EDGE('',*,*,#2824,.F.);
#3560=ORIENTED_EDGE('',*,*,#2821,.F.);
#3561=ORIENTED_EDGE('',*,*,#2817,.T.);
#3562=ORIENTED_EDGE('',*,*,#2822,.T.);
#3563=ORIENTED_EDGE('',*,*,#2824,.T.);
#3564=ORIENTED_EDGE('',*,*,#2818,.T.);
#3565=ORIENTED_EDGE('',*,*,#2802,.T.);
#3566=ORIENTED_EDGE('',*,*,#2811,.T.);
#3567=ORIENTED_EDGE('',*,*,#2808,.T.);
#3568=ORIENTED_EDGE('',*,*,#2804,.T.);
#3569=ORIENTED_EDGE('',*,*,#2798,.T.);
#3570=ORIENTED_EDGE('',*,*,#2794,.F.);
#3571=ORIENTED_EDGE('',*,*,#2815,.T.);
#3572=ORIENTED_EDGE('',*,*,#2820,.T.);
#3573=ORIENTED_EDGE('',*,*,#2823,.T.);
#3574=ORIENTED_EDGE('',*,*,#2825,.F.);
#3575=ORIENTED_EDGE('',*,*,#2826,.T.);
#3576=ORIENTED_EDGE('',*,*,#2827,.F.);
#3577=ORIENTED_EDGE('',*,*,#2826,.F.);
#3578=ORIENTED_EDGE('',*,*,#2828,.F.);
#3579=ORIENTED_EDGE('',*,*,#2829,.F.);
#3580=ORIENTED_EDGE('',*,*,#2830,.T.);
#3581=ORIENTED_EDGE('',*,*,#2831,.T.);
#3582=ORIENTED_EDGE('',*,*,#2832,.T.);
#3583=ORIENTED_EDGE('',*,*,#2833,.T.);
#3584=ORIENTED_EDGE('',*,*,#2827,.T.);
#3585=ORIENTED_EDGE('',*,*,#2834,.F.);
#3586=ORIENTED_EDGE('',*,*,#2835,.F.);
#3587=ORIENTED_EDGE('',*,*,#2836,.T.);
#3588=ORIENTED_EDGE('',*,*,#2830,.F.);
#3589=ORIENTED_EDGE('',*,*,#2837,.F.);
#3590=ORIENTED_EDGE('',*,*,#2833,.F.);
#3591=ORIENTED_EDGE('',*,*,#2838,.F.);
#3592=ORIENTED_EDGE('',*,*,#2839,.F.);
#3593=ORIENTED_EDGE('',*,*,#2840,.F.);
#3594=ORIENTED_EDGE('',*,*,#2838,.T.);
#3595=ORIENTED_EDGE('',*,*,#2832,.F.);
#3596=ORIENTED_EDGE('',*,*,#2841,.F.);
#3597=ORIENTED_EDGE('',*,*,#2842,.F.);
#3598=ORIENTED_EDGE('',*,*,#2841,.T.);
#3599=ORIENTED_EDGE('',*,*,#2831,.F.);
#3600=ORIENTED_EDGE('',*,*,#2836,.F.);
#3601=ORIENTED_EDGE('',*,*,#2839,.T.);
#3602=ORIENTED_EDGE('',*,*,#2840,.T.);
#3603=ORIENTED_EDGE('',*,*,#2842,.T.);
#3604=ORIENTED_EDGE('',*,*,#2835,.T.);
#3605=ORIENTED_EDGE('',*,*,#2843,.T.);
#3606=ORIENTED_EDGE('',*,*,#2844,.T.);
#3607=ORIENTED_EDGE('',*,*,#2845,.T.);
#3608=ORIENTED_EDGE('',*,*,#2846,.T.);
#3609=ORIENTED_EDGE('',*,*,#2825,.T.);
#3610=ORIENTED_EDGE('',*,*,#2789,.F.);
#3611=ORIENTED_EDGE('',*,*,#2847,.F.);
#3612=ORIENTED_EDGE('',*,*,#2844,.F.);
#3613=ORIENTED_EDGE('',*,*,#2848,.T.);
#3614=ORIENTED_EDGE('',*,*,#2849,.F.);
#3615=ORIENTED_EDGE('',*,*,#2788,.F.);
#3616=ORIENTED_EDGE('',*,*,#2850,.F.);
#3617=ORIENTED_EDGE('',*,*,#2845,.F.);
#3618=ORIENTED_EDGE('',*,*,#2847,.T.);
#3619=ORIENTED_EDGE('',*,*,#2837,.T.);
#3620=ORIENTED_EDGE('',*,*,#2846,.F.);
#3621=ORIENTED_EDGE('',*,*,#2850,.T.);
#3622=ORIENTED_EDGE('',*,*,#2791,.F.);
#3623=ORIENTED_EDGE('',*,*,#2851,.F.);
#3624=ORIENTED_EDGE('',*,*,#2852,.F.);
#3625=ORIENTED_EDGE('',*,*,#2828,.T.);
#3626=ORIENTED_EDGE('',*,*,#2829,.T.);
#3627=ORIENTED_EDGE('',*,*,#2852,.T.);
#3628=ORIENTED_EDGE('',*,*,#2853,.F.);
#3629=ORIENTED_EDGE('',*,*,#2848,.F.);
#3630=ORIENTED_EDGE('',*,*,#2843,.F.);
#3631=ORIENTED_EDGE('',*,*,#2834,.T.);
#3632=ORIENTED_EDGE('',*,*,#2790,.F.);
#3633=ORIENTED_EDGE('',*,*,#2849,.T.);
#3634=ORIENTED_EDGE('',*,*,#2853,.T.);
#3635=ORIENTED_EDGE('',*,*,#2851,.T.);
#3636=ORIENTED_EDGE('',*,*,#2854,.F.);
#3637=ORIENTED_EDGE('',*,*,#2855,.T.);
#3638=ORIENTED_EDGE('',*,*,#2723,.T.);
#3639=ORIENTED_EDGE('',*,*,#2855,.F.);
#3640=ORIENTED_EDGE('',*,*,#2856,.F.);
#3641=ORIENTED_EDGE('',*,*,#2857,.T.);
#3642=ORIENTED_EDGE('',*,*,#2729,.T.);
#3643=ORIENTED_EDGE('',*,*,#2857,.F.);
#3644=ORIENTED_EDGE('',*,*,#2858,.F.);
#3645=ORIENTED_EDGE('',*,*,#2859,.T.);
#3646=ORIENTED_EDGE('',*,*,#2735,.T.);
#3647=ORIENTED_EDGE('',*,*,#2859,.F.);
#3648=ORIENTED_EDGE('',*,*,#2860,.F.);
#3649=ORIENTED_EDGE('',*,*,#2861,.T.);
#3650=ORIENTED_EDGE('',*,*,#2741,.T.);
#3651=ORIENTED_EDGE('',*,*,#2861,.F.);
#3652=ORIENTED_EDGE('',*,*,#2862,.F.);
#3653=ORIENTED_EDGE('',*,*,#2863,.T.);
#3654=ORIENTED_EDGE('',*,*,#2864,.F.);
#3655=ORIENTED_EDGE('',*,*,#2865,.T.);
#3656=ORIENTED_EDGE('',*,*,#2862,.T.);
#3657=ORIENTED_EDGE('',*,*,#2865,.F.);
#3658=ORIENTED_EDGE('',*,*,#2864,.T.);
#3659=ORIENTED_EDGE('',*,*,#2787,.T.);
#3660=ORIENTED_EDGE('',*,*,#2863,.F.);
#3661=ORIENTED_EDGE('',*,*,#2866,.T.);
#3662=ORIENTED_EDGE('',*,*,#2750,.F.);
#3663=ORIENTED_EDGE('',*,*,#2866,.F.);
#3664=ORIENTED_EDGE('',*,*,#2752,.F.);
#3665=ORIENTED_EDGE('',*,*,#2854,.T.);
#3666=ORIENTED_EDGE('',*,*,#2856,.T.);
#3667=ORIENTED_EDGE('',*,*,#2858,.T.);
#3668=ORIENTED_EDGE('',*,*,#2860,.T.);
#4501=CYLINDRICAL_SURFACE('',#5263,0.5);
#4502=CYLINDRICAL_SURFACE('',#5269,0.5);
#4503=CYLINDRICAL_SURFACE('',#5275,0.5);
#4504=CYLINDRICAL_SURFACE('',#5281,0.5);
#4505=CYLINDRICAL_SURFACE('',#5290,1.8);
#4506=CYLINDRICAL_SURFACE('',#5292,0.3);
#4507=CYLINDRICAL_SURFACE('',#5309,0.5);
#4508=CYLINDRICAL_SURFACE('',#5315,0.305);
#4509=CYLINDRICAL_SURFACE('',#5329,0.305);
#4510=CYLINDRICAL_SURFACE('',#5343,0.275);
#4511=CYLINDRICAL_SURFACE('',#5345,0.275);
#4512=CYLINDRICAL_SURFACE('',#5347,0.275);
#4513=CYLINDRICAL_SURFACE('',#5349,0.275);
#4514=CYLINDRICAL_SURFACE('',#5354,0.7);
#4515=CYLINDRICAL_SURFACE('',#5357,0.5);
#4614=ADVANCED_FACE('',(#659,#366),#476,.T.);
#4615=ADVANCED_FACE('',(#660),#4501,.F.);
#4616=ADVANCED_FACE('',(#661,#367),#477,.T.);
#4617=ADVANCED_FACE('',(#662),#4502,.F.);
#4618=ADVANCED_FACE('',(#663,#368),#478,.T.);
#4619=ADVANCED_FACE('',(#664),#4503,.F.);
#4620=ADVANCED_FACE('',(#665,#369),#479,.T.);
#4621=ADVANCED_FACE('',(#666),#4504,.F.);
#4622=ADVANCED_FACE('',(#667,#370),#480,.T.);
#4623=ADVANCED_FACE('',(#668),#4505,.T.);
#4624=ADVANCED_FACE('',(#669),#4506,.T.);
#4625=ADVANCED_FACE('',(#670),#481,.T.);
#4626=ADVANCED_FACE('',(#671,#371),#482,.T.);
#4627=ADVANCED_FACE('',(#672),#483,.T.);
#4628=ADVANCED_FACE('',(#673),#484,.T.);
#4629=ADVANCED_FACE('',(#674),#485,.T.);
#4630=ADVANCED_FACE('',(#675),#486,.T.);
#4631=ADVANCED_FACE('',(#676),#487,.T.);
#4632=ADVANCED_FACE('',(#677),#488,.T.);
#4633=ADVANCED_FACE('',(#678),#489,.T.);
#4634=ADVANCED_FACE('',(#679),#490,.T.);
#4635=ADVANCED_FACE('',(#680),#491,.T.);
#4636=ADVANCED_FACE('',(#681),#492,.F.);
#4637=ADVANCED_FACE('',(#682,#372,#373),#4507,.T.);
#4638=ADVANCED_FACE('',(#683),#4508,.F.);
#4639=ADVANCED_FACE('',(#684),#493,.T.);
#4640=ADVANCED_FACE('',(#685),#494,.T.);
#4641=ADVANCED_FACE('',(#686),#495,.T.);
#4642=ADVANCED_FACE('',(#687),#496,.T.);
#4643=ADVANCED_FACE('',(#688,#374),#497,.F.);
#4644=ADVANCED_FACE('',(#689),#498,.T.);
#4645=ADVANCED_FACE('',(#690),#499,.T.);
#4646=ADVANCED_FACE('',(#691),#500,.T.);
#4647=ADVANCED_FACE('',(#692),#501,.T.);
#4648=ADVANCED_FACE('',(#693,#375),#502,.T.);
#4649=ADVANCED_FACE('',(#694),#503,.F.);
#4650=ADVANCED_FACE('',(#695),#4509,.F.);
#4651=ADVANCED_FACE('',(#696,#376),#504,.T.);
#4652=ADVANCED_FACE('',(#697),#505,.T.);
#4653=ADVANCED_FACE('',(#698),#506,.T.);
#4654=ADVANCED_FACE('',(#699),#507,.T.);
#4655=ADVANCED_FACE('',(#700),#508,.T.);
#4656=ADVANCED_FACE('',(#701,#377),#509,.F.);
#4657=ADVANCED_FACE('',(#702),#510,.T.);
#4658=ADVANCED_FACE('',(#703),#511,.T.);
#4659=ADVANCED_FACE('',(#704),#512,.T.);
#4660=ADVANCED_FACE('',(#705),#513,.T.);
#4661=ADVANCED_FACE('',(#706),#514,.T.);
#4662=ADVANCED_FACE('',(#707),#4510,.F.);
#4663=ADVANCED_FACE('',(#708),#4511,.F.);
#4664=ADVANCED_FACE('',(#709),#4512,.F.);
#4665=ADVANCED_FACE('',(#710),#4513,.F.);
#4666=ADVANCED_FACE('',(#711,#378),#515,.F.);
#4667=ADVANCED_FACE('',(#712),#4514,.T.);
#4668=ADVANCED_FACE('',(#713,#379),#516,.T.);
#4669=ADVANCED_FACE('',(#714),#4515,.T.);
#4670=ADVANCED_FACE('',(#715,#380,#381,#382,#383),#517,.F.);
#4902=CLOSED_SHELL('',(#4614,#4615,#4616,#4617,#4618,#4619,#4620,#4621,
#4622,#4623,#4624,#4625,#4626,#4627,#4628,#4629,#4630,#4631,#4632,#4633,
#4634,#4635,#4636,#4637,#4638,#4639,#4640,#4641,#4642,#4643,#4644,#4645,
#4646,#4647,#4648,#4649,#4650,#4651,#4652,#4653,#4654,#4655,#4656,#4657,
#4658,#4659,#4660,#4661,#4662,#4663,#4664,#4665,#4666,#4667,#4668,#4669,
#4670));
#5258=AXIS2_PLACEMENT_3D('',#7593,#5980,#5981);
#5259=AXIS2_PLACEMENT_3D('',#7594,#5982,#5983);
#5260=AXIS2_PLACEMENT_3D('',#7597,#5984,#5985);
#5261=AXIS2_PLACEMENT_3D('',#7598,#5986,#5987);
#5262=AXIS2_PLACEMENT_3D('',#7600,#5988,#5989);
#5263=AXIS2_PLACEMENT_3D('',#7601,#5990,#5991);
#5264=AXIS2_PLACEMENT_3D('',#7605,#5993,#5994);
#5265=AXIS2_PLACEMENT_3D('',#7607,#5996,#5997);
#5266=AXIS2_PLACEMENT_3D('',#7610,#5998,#5999);
#5267=AXIS2_PLACEMENT_3D('',#7611,#6000,#6001);
#5268=AXIS2_PLACEMENT_3D('',#7613,#6002,#6003);
#5269=AXIS2_PLACEMENT_3D('',#7614,#6004,#6005);
#5270=AXIS2_PLACEMENT_3D('',#7618,#6007,#6008);
#5271=AXIS2_PLACEMENT_3D('',#7620,#6010,#6011);
#5272=AXIS2_PLACEMENT_3D('',#7623,#6012,#6013);
#5273=AXIS2_PLACEMENT_3D('',#7624,#6014,#6015);
#5274=AXIS2_PLACEMENT_3D('',#7626,#6016,#6017);
#5275=AXIS2_PLACEMENT_3D('',#7627,#6018,#6019);
#5276=AXIS2_PLACEMENT_3D('',#7631,#6021,#6022);
#5277=AXIS2_PLACEMENT_3D('',#7633,#6024,#6025);
#5278=AXIS2_PLACEMENT_3D('',#7636,#6026,#6027);
#5279=AXIS2_PLACEMENT_3D('',#7637,#6028,#6029);
#5280=AXIS2_PLACEMENT_3D('',#7639,#6030,#6031);
#5281=AXIS2_PLACEMENT_3D('',#7640,#6032,#6033);
#5282=AXIS2_PLACEMENT_3D('',#7644,#6035,#6036);
#5283=AXIS2_PLACEMENT_3D('',#7646,#6038,#6039);
#5284=AXIS2_PLACEMENT_3D('',#7647,#6040,#6041);
#5285=AXIS2_PLACEMENT_3D('',#7648,#6042,#6043);
#5286=AXIS2_PLACEMENT_3D('',#7649,#6044,#6045);
#5287=AXIS2_PLACEMENT_3D('',#7651,#6046,#6047);
#5288=AXIS2_PLACEMENT_3D('',#7652,#6048,#6049);
#5289=AXIS2_PLACEMENT_3D('',#7654,#6050,#6051);
#5290=AXIS2_PLACEMENT_3D('',#7655,#6052,#6053);
#5291=AXIS2_PLACEMENT_3D('',#7658,#6055,#6056);
#5292=AXIS2_PLACEMENT_3D('',#7659,#6057,#6058);
#5293=AXIS2_PLACEMENT_3D('',#7661,#6059,#6060);
#5294=AXIS2_PLACEMENT_3D('',#7664,#6062,#6063);
#5295=AXIS2_PLACEMENT_3D('',#7665,#6064,#6065);
#5296=AXIS2_PLACEMENT_3D('',#7666,#6066,#6067);
#5297=AXIS2_PLACEMENT_3D('',#7679,#6074,#6075);
#5298=AXIS2_PLACEMENT_3D('',#7685,#6079,#6080);
#5299=AXIS2_PLACEMENT_3D('',#7691,#6084,#6085);
#5300=AXIS2_PLACEMENT_3D('',#7693,#6087,#6088);
#5301=AXIS2_PLACEMENT_3D('',#7699,#6092,#6093);
#5302=AXIS2_PLACEMENT_3D('',#7707,#6097,#6098);
#5303=AXIS2_PLACEMENT_3D('',#7709,#6100,#6101);
#5304=AXIS2_PLACEMENT_3D('',#7713,#6104,#6105);
#5305=AXIS2_PLACEMENT_3D('',#7719,#6109,#6110);
#5306=AXIS2_PLACEMENT_3D('',#7723,#6113,#6114);
#5307=AXIS2_PLACEMENT_3D('',#7725,#6116,#6117);
#5308=AXIS2_PLACEMENT_3D('',#7726,#6118,#6119);
#5309=AXIS2_PLACEMENT_3D('',#7727,#6120,#6121);
#5310=AXIS2_PLACEMENT_3D('',#7730,#6123,#6124);
#5311=AXIS2_PLACEMENT_3D('',#7735,#6126,#6127);
#5312=AXIS2_PLACEMENT_3D('',#7738,#6129,#6130);
#5313=AXIS2_PLACEMENT_3D('',#7743,#6132,#6133);
#5314=AXIS2_PLACEMENT_3D('',#7746,#6135,#6136);
#5315=AXIS2_PLACEMENT_3D('',#7747,#6137,#6138);
#5316=AXIS2_PLACEMENT_3D('',#7749,#6139,#6140);
#5317=AXIS2_PLACEMENT_3D('',#7752,#6142,#6143);
#5318=AXIS2_PLACEMENT_3D('',#7753,#6144,#6145);
#5319=AXIS2_PLACEMENT_3D('',#7762,#6150,#6151);
#5320=AXIS2_PLACEMENT_3D('',#7771,#6156,#6157);
#5321=AXIS2_PLACEMENT_3D('',#7777,#6161,#6162);
#5322=AXIS2_PLACEMENT_3D('',#7780,#6165,#6166);
#5323=AXIS2_PLACEMENT_3D('',#7784,#6169,#6170);
#5324=AXIS2_PLACEMENT_3D('',#7791,#6175,#6176);
#5325=AXIS2_PLACEMENT_3D('',#7797,#6180,#6181);
#5326=AXIS2_PLACEMENT_3D('',#7801,#6184,#6185);
#5327=AXIS2_PLACEMENT_3D('',#7804,#6188,#6189);
#5328=AXIS2_PLACEMENT_3D('',#7805,#6190,#6191);
#5329=AXIS2_PLACEMENT_3D('',#7806,#6192,#6193);
#5330=AXIS2_PLACEMENT_3D('',#7808,#6194,#6195);
#5331=AXIS2_PLACEMENT_3D('',#7811,#6197,#6198);
#5332=AXIS2_PLACEMENT_3D('',#7812,#6199,#6200);
#5333=AXIS2_PLACEMENT_3D('',#7825,#6207,#6208);
#5334=AXIS2_PLACEMENT_3D('',#7831,#6212,#6213);
#5335=AXIS2_PLACEMENT_3D('',#7837,#6217,#6218);
#5336=AXIS2_PLACEMENT_3D('',#7841,#6221,#6222);
#5337=AXIS2_PLACEMENT_3D('',#7843,#6224,#6225);
#5338=AXIS2_PLACEMENT_3D('',#7851,#6230,#6231);
#5339=AXIS2_PLACEMENT_3D('',#7856,#6235,#6236);
#5340=AXIS2_PLACEMENT_3D('',#7858,#6238,#6239);
#5341=AXIS2_PLACEMENT_3D('',#7862,#6242,#6243);
#5342=AXIS2_PLACEMENT_3D('',#7864,#6245,#6246);
#5343=AXIS2_PLACEMENT_3D('',#7865,#6247,#6248);
#5344=AXIS2_PLACEMENT_3D('',#7867,#6249,#6250);
#5345=AXIS2_PLACEMENT_3D('',#7869,#6252,#6253);
#5346=AXIS2_PLACEMENT_3D('',#7871,#6254,#6255);
#5347=AXIS2_PLACEMENT_3D('',#7873,#6257,#6258);
#5348=AXIS2_PLACEMENT_3D('',#7875,#6259,#6260);
#5349=AXIS2_PLACEMENT_3D('',#7877,#6262,#6263);
#5350=AXIS2_PLACEMENT_3D('',#7879,#6264,#6265);
#5351=AXIS2_PLACEMENT_3D('',#7881,#6267,#6268);
#5352=AXIS2_PLACEMENT_3D('',#7883,#6269,#6270);
#5353=AXIS2_PLACEMENT_3D('',#7885,#6271,#6272);
#5354=AXIS2_PLACEMENT_3D('',#7886,#6273,#6274);
#5355=AXIS2_PLACEMENT_3D('',#7888,#6275,#6276);
#5356=AXIS2_PLACEMENT_3D('',#7890,#6278,#6279);
#5357=AXIS2_PLACEMENT_3D('',#7891,#6280,#6281);
#5358=AXIS2_PLACEMENT_3D('',#7893,#6283,#6284);
#5980=DIRECTION('axis',(0.,0.,1.));
#5981=DIRECTION('refdir',(1.,0.,0.));
#5982=DIRECTION('center_axis',(0.,0.,1.));
#5983=DIRECTION('ref_axis',(1.,0.,0.));
#5984=DIRECTION('center_axis',(0.,0.,-1.));
#5985=DIRECTION('ref_axis',(1.,0.,0.));
#5986=DIRECTION('center_axis',(0.,0.,1.));
#5987=DIRECTION('ref_axis',(1.,0.,0.));
#5988=DIRECTION('center_axis',(0.,0.,1.));
#5989=DIRECTION('ref_axis',(1.,0.,0.));
#5990=DIRECTION('center_axis',(0.,0.,1.));
#5991=DIRECTION('ref_axis',(0.707106781186548,0.707106781186547,0.));
#5992=DIRECTION('',(0.,0.,-1.));
#5993=DIRECTION('center_axis',(0.,0.,-1.));
#5994=DIRECTION('ref_axis',(1.,0.,0.));
#5995=DIRECTION('',(0.,0.,1.));
#5996=DIRECTION('center_axis',(0.,0.,1.));
#5997=DIRECTION('ref_axis',(1.,0.,0.));
#5998=DIRECTION('center_axis',(0.,0.,-1.));
#5999=DIRECTION('ref_axis',(1.,0.,0.));
#6000=DIRECTION('center_axis',(0.,0.,1.));
#6001=DIRECTION('ref_axis',(1.,0.,0.));
#6002=DIRECTION('center_axis',(0.,0.,1.));
#6003=DIRECTION('ref_axis',(1.,0.,0.));
#6004=DIRECTION('center_axis',(0.,0.,1.));
#6005=DIRECTION('ref_axis',(0.707106781186547,-0.707106781186548,0.));
#6006=DIRECTION('',(0.,0.,-1.));
#6007=DIRECTION('center_axis',(0.,0.,-1.));
#6008=DIRECTION('ref_axis',(1.,0.,0.));
#6009=DIRECTION('',(0.,0.,1.));
#6010=DIRECTION('center_axis',(0.,0.,1.));
#6011=DIRECTION('ref_axis',(1.,0.,0.));
#6012=DIRECTION('center_axis',(0.,0.,-1.));
#6013=DIRECTION('ref_axis',(1.,0.,0.));
#6014=DIRECTION('center_axis',(0.,0.,1.));
#6015=DIRECTION('ref_axis',(1.,0.,0.));
#6016=DIRECTION('center_axis',(0.,0.,1.));
#6017=DIRECTION('ref_axis',(1.,0.,0.));
#6018=DIRECTION('center_axis',(0.,0.,1.));
#6019=DIRECTION('ref_axis',(-0.707106781186548,-0.707106781186547,0.));
#6020=DIRECTION('',(0.,0.,-1.));
#6021=DIRECTION('center_axis',(0.,0.,-1.));
#6022=DIRECTION('ref_axis',(1.,0.,0.));
#6023=DIRECTION('',(0.,0.,1.));
#6024=DIRECTION('center_axis',(0.,0.,1.));
#6025=DIRECTION('ref_axis',(1.,0.,0.));
#6026=DIRECTION('center_axis',(0.,0.,-1.));
#6027=DIRECTION('ref_axis',(1.,0.,0.));
#6028=DIRECTION('center_axis',(0.,0.,1.));
#6029=DIRECTION('ref_axis',(1.,0.,0.));
#6030=DIRECTION('center_axis',(0.,0.,1.));
#6031=DIRECTION('ref_axis',(1.,0.,0.));
#6032=DIRECTION('center_axis',(0.,0.,1.));
#6033=DIRECTION('ref_axis',(-0.707106781186547,0.707106781186548,0.));
#6034=DIRECTION('',(0.,0.,-1.));
#6035=DIRECTION('center_axis',(0.,0.,-1.));
#6036=DIRECTION('ref_axis',(1.,0.,0.));
#6037=DIRECTION('',(0.,0.,1.));
#6038=DIRECTION('center_axis',(0.,0.,1.));
#6039=DIRECTION('ref_axis',(1.,0.,0.));
#6040=DIRECTION('center_axis',(0.,0.,1.));
#6041=DIRECTION('ref_axis',(1.,0.,0.));
#6042=DIRECTION('center_axis',(0.,0.,1.));
#6043=DIRECTION('ref_axis',(1.,0.,0.));
#6044=DIRECTION('center_axis',(0.,0.,1.));
#6045=DIRECTION('ref_axis',(1.,0.,0.));
#6046=DIRECTION('center_axis',(0.,0.,1.));
#6047=DIRECTION('ref_axis',(1.,0.,0.));
#6048=DIRECTION('center_axis',(0.,0.,1.));
#6049=DIRECTION('ref_axis',(1.,0.,0.));
#6050=DIRECTION('center_axis',(0.,0.,-1.));
#6051=DIRECTION('ref_axis',(1.,0.,0.));
#6052=DIRECTION('center_axis',(0.,0.,1.));
#6053=DIRECTION('ref_axis',(1.,0.,0.));
#6054=DIRECTION('',(0.,0.,-1.));
#6055=DIRECTION('center_axis',(0.,0.,1.));
#6056=DIRECTION('ref_axis',(1.,0.,0.));
#6057=DIRECTION('center_axis',(0.,1.,0.));
#6058=DIRECTION('ref_axis',(1.,0.,0.));
#6059=DIRECTION('center_axis',(0.,1.,0.));
#6060=DIRECTION('ref_axis',(1.,0.,0.));
#6061=DIRECTION('',(0.,-1.,0.));
#6062=DIRECTION('center_axis',(0.,-1.,0.));
#6063=DIRECTION('ref_axis',(1.,0.,0.));
#6064=DIRECTION('center_axis',(0.,1.,0.));
#6065=DIRECTION('ref_axis',(1.,0.,0.));
#6066=DIRECTION('center_axis',(0.,1.,0.));
#6067=DIRECTION('ref_axis',(0.,0.,1.));
#6068=DIRECTION('',(0.,0.,1.));
#6069=DIRECTION('',(-1.,0.,0.));
#6070=DIRECTION('',(0.,0.,-1.));
#6071=DIRECTION('',(-1.,0.,0.));
#6072=DIRECTION('',(0.,0.,1.));
#6073=DIRECTION('',(1.,0.,0.));
#6074=DIRECTION('center_axis',(1.,0.,0.));
#6075=DIRECTION('ref_axis',(0.,0.,-1.));
#6076=DIRECTION('',(0.,1.,0.));
#6077=DIRECTION('',(0.,0.,1.));
#6078=DIRECTION('',(0.,1.,0.));
#6079=DIRECTION('center_axis',(-1.,0.,0.));
#6080=DIRECTION('ref_axis',(0.,0.,1.));
#6081=DIRECTION('',(0.,0.,-1.));
#6082=DIRECTION('',(0.,1.,0.));
#6083=DIRECTION('',(0.,1.,0.));
#6084=DIRECTION('center_axis',(0.,0.,-1.));
#6085=DIRECTION('ref_axis',(-1.,0.,0.));
#6086=DIRECTION('',(1.,0.,0.));
#6087=DIRECTION('center_axis',(-1.,0.,0.));
#6088=DIRECTION('ref_axis',(0.,-1.,0.));
#6089=DIRECTION('',(0.,-1.,0.));
#6090=DIRECTION('',(0.,0.,1.));
#6091=DIRECTION('',(0.,-1.,0.));
#6092=DIRECTION('center_axis',(0.,0.,1.));
#6093=DIRECTION('ref_axis',(1.,0.,0.));
#6094=DIRECTION('',(-1.,0.,0.));
#6095=DIRECTION('',(0.,1.,0.));
#6096=DIRECTION('',(-1.,0.,0.));
#6097=DIRECTION('center_axis',(0.,0.,1.));
#6098=DIRECTION('ref_axis',(1.,0.,0.));
#6099=DIRECTION('',(-1.,0.,0.));
#6100=DIRECTION('center_axis',(0.,1.,0.));
#6101=DIRECTION('ref_axis',(-1.,0.,0.));
#6102=DIRECTION('',(0.,0.,1.));
#6103=DIRECTION('',(-1.,0.,0.));
#6104=DIRECTION('center_axis',(0.,1.,0.));
#6105=DIRECTION('ref_axis',(-1.,0.,0.));
#6106=DIRECTION('',(0.,0.,-1.));
#6107=DIRECTION('',(0.,0.,1.));
#6108=DIRECTION('',(-1.,0.,0.));
#6109=DIRECTION('center_axis',(1.,0.,0.));
#6110=DIRECTION('ref_axis',(0.,1.,0.));
#6111=DIRECTION('',(0.,1.,0.));
#6112=DIRECTION('',(0.,0.,1.));
#6113=DIRECTION('center_axis',(0.,-1.,0.));
#6114=DIRECTION('ref_axis',(1.,0.,0.));
#6115=DIRECTION('',(1.,0.,0.));
#6116=DIRECTION('center_axis',(0.,0.,1.));
#6117=DIRECTION('ref_axis',(1.,0.,0.));
#6118=DIRECTION('center_axis',(0.,0.,-1.));
#6119=DIRECTION('ref_axis',(1.,0.,0.));
#6120=DIRECTION('center_axis',(0.,0.,1.));
#6121=DIRECTION('ref_axis',(1.,0.,0.));
#6122=DIRECTION('',(0.,0.,-1.));
#6123=DIRECTION('center_axis',(0.,0.,-1.));
#6124=DIRECTION('ref_axis',(1.,0.,0.));
#6125=DIRECTION('',(0.,0.,1.));
#6126=DIRECTION('center_axis',(0.,0.,1.));
#6127=DIRECTION('ref_axis',(1.,0.,0.));
#6128=DIRECTION('',(0.,0.,-1.));
#6129=DIRECTION('center_axis',(0.,0.,-1.));
#6130=DIRECTION('ref_axis',(1.,0.,0.));
#6131=DIRECTION('',(0.,0.,-1.));
#6132=DIRECTION('center_axis',(0.,0.,-1.));
#6133=DIRECTION('ref_axis',(1.,0.,0.));
#6134=DIRECTION('',(0.,0.,1.));
#6135=DIRECTION('center_axis',(0.,0.,1.));
#6136=DIRECTION('ref_axis',(1.,0.,0.));
#6137=DIRECTION('center_axis',(0.,1.,0.));
#6138=DIRECTION('ref_axis',(1.,0.,0.));
#6139=DIRECTION('center_axis',(0.,1.,0.));
#6140=DIRECTION('ref_axis',(1.,0.,0.));
#6141=DIRECTION('',(0.,1.,0.));
#6142=DIRECTION('center_axis',(0.,-1.,0.));
#6143=DIRECTION('ref_axis',(1.,0.,0.));
#6144=DIRECTION('center_axis',(0.,0.,1.));
#6145=DIRECTION('ref_axis',(1.,0.,0.));
#6146=DIRECTION('',(0.,1.,0.));
#6147=DIRECTION('',(-1.,0.,0.));
#6148=DIRECTION('',(0.,1.,0.));
#6149=DIRECTION('',(1.,0.,0.));
#6150=DIRECTION('center_axis',(-1.,0.,0.));
#6151=DIRECTION('ref_axis',(0.,0.,1.));
#6152=DIRECTION('',(0.,-1.,0.));
#6153=DIRECTION('',(0.,0.,1.));
#6154=DIRECTION('',(0.,1.,0.));
#6155=DIRECTION('',(0.,0.,-1.));
#6156=DIRECTION('center_axis',(0.,0.,-1.));
#6157=DIRECTION('ref_axis',(-1.,0.,0.));
#6158=DIRECTION('',(1.,0.,0.));
#6159=DIRECTION('',(-1.,0.,0.));
#6160=DIRECTION('',(0.,1.,0.));
#6161=DIRECTION('center_axis',(1.,0.,0.));
#6162=DIRECTION('ref_axis',(0.,0.,-1.));
#6163=DIRECTION('',(0.,0.,1.));
#6164=DIRECTION('',(0.,0.,-1.));
#6165=DIRECTION('center_axis',(0.,1.,0.));
#6166=DIRECTION('ref_axis',(1.,0.,0.));
#6167=DIRECTION('',(1.,0.,0.));
#6168=DIRECTION('',(0.,0.,1.));
#6169=DIRECTION('center_axis',(0.,0.,-1.));
#6170=DIRECTION('ref_axis',(-1.,0.,0.));
#6171=DIRECTION('',(0.,1.,0.));
#6172=DIRECTION('',(1.,0.,0.));
#6173=DIRECTION('',(0.,1.,0.));
#6174=DIRECTION('',(-1.,0.,0.));
#6175=DIRECTION('center_axis',(1.,0.,0.));
#6176=DIRECTION('ref_axis',(0.,0.,-1.));
#6177=DIRECTION('',(0.,0.,-1.));
#6178=DIRECTION('',(0.,1.,0.));
#6179=DIRECTION('',(0.,0.,1.));
#6180=DIRECTION('center_axis',(-1.,0.,0.));
#6181=DIRECTION('ref_axis',(0.,0.,1.));
#6182=DIRECTION('',(0.,1.,0.));
#6183=DIRECTION('',(0.,0.,1.));
#6184=DIRECTION('center_axis',(0.,0.,1.));
#6185=DIRECTION('ref_axis',(1.,0.,0.));
#6186=DIRECTION('',(-1.,0.,0.));
#6187=DIRECTION('',(1.,0.,0.));
#6188=DIRECTION('center_axis',(0.,1.,0.));
#6189=DIRECTION('ref_axis',(0.,0.,1.));
#6190=DIRECTION('center_axis',(0.,1.,0.));
#6191=DIRECTION('ref_axis',(1.,0.,0.));
#6192=DIRECTION('center_axis',(0.,1.,0.));
#6193=DIRECTION('ref_axis',(1.,0.,0.));
#6194=DIRECTION('center_axis',(0.,1.,0.));
#6195=DIRECTION('ref_axis',(1.,0.,0.));
#6196=DIRECTION('',(0.,1.,0.));
#6197=DIRECTION('center_axis',(0.,-1.,0.));
#6198=DIRECTION('ref_axis',(1.,0.,0.));
#6199=DIRECTION('center_axis',(0.,1.,0.));
#6200=DIRECTION('ref_axis',(0.,0.,1.));
#6201=DIRECTION('',(-1.,0.,0.));
#6202=DIRECTION('',(0.,0.,-1.));
#6203=DIRECTION('',(1.,0.,0.));
#6204=DIRECTION('',(0.,0.,-1.));
#6205=DIRECTION('',(-1.,0.,0.));
#6206=DIRECTION('',(0.,0.,1.));
#6207=DIRECTION('center_axis',(0.,0.,1.));
#6208=DIRECTION('ref_axis',(1.,0.,0.));
#6209=DIRECTION('',(0.,1.,0.));
#6210=DIRECTION('',(-1.,0.,0.));
#6211=DIRECTION('',(0.,1.,0.));
#6212=DIRECTION('center_axis',(-1.,0.,0.));
#6213=DIRECTION('ref_axis',(0.,0.,1.));
#6214=DIRECTION('',(0.,-1.,0.));
#6215=DIRECTION('',(0.,1.,0.));
#6216=DIRECTION('',(0.,0.,-1.));
#6217=DIRECTION('center_axis',(0.,0.,-1.));
#6218=DIRECTION('ref_axis',(-1.,0.,0.));
#6219=DIRECTION('',(1.,0.,0.));
#6220=DIRECTION('',(0.,1.,0.));
#6221=DIRECTION('center_axis',(1.,0.,0.));
#6222=DIRECTION('ref_axis',(0.,0.,-1.));
#6223=DIRECTION('',(0.,0.,1.));
#6224=DIRECTION('center_axis',(0.,1.,0.));
#6225=DIRECTION('ref_axis',(1.,0.,0.));
#6226=DIRECTION('',(0.,0.,1.));
#6227=DIRECTION('',(-1.,0.,0.));
#6228=DIRECTION('',(0.,0.,-1.));
#6229=DIRECTION('',(1.,0.,0.));
#6230=DIRECTION('center_axis',(0.,0.,1.));
#6231=DIRECTION('ref_axis',(1.,0.,0.));
#6232=DIRECTION('',(0.,1.,0.));
#6233=DIRECTION('',(0.,1.,0.));
#6234=DIRECTION('',(1.,0.,0.));
#6235=DIRECTION('center_axis',(-1.,0.,0.));
#6236=DIRECTION('ref_axis',(0.,0.,1.));
#6237=DIRECTION('',(0.,1.,0.));
#6238=DIRECTION('center_axis',(0.,0.,-1.));
#6239=DIRECTION('ref_axis',(-1.,0.,0.));
#6240=DIRECTION('',(-1.,0.,0.));
#6241=DIRECTION('',(0.,1.,0.));
#6242=DIRECTION('center_axis',(1.,0.,0.));
#6243=DIRECTION('ref_axis',(0.,0.,-1.));
#6244=DIRECTION('',(0.,0.,-1.));
#6245=DIRECTION('center_axis',(0.,1.,0.));
#6246=DIRECTION('ref_axis',(0.,0.,1.));
#6247=DIRECTION('center_axis',(0.,0.,1.));
#6248=DIRECTION('ref_axis',(1.,0.,0.));
#6249=DIRECTION('center_axis',(0.,0.,1.));
#6250=DIRECTION('ref_axis',(1.,0.,0.));
#6251=DIRECTION('',(0.,0.,1.));
#6252=DIRECTION('center_axis',(0.,0.,1.));
#6253=DIRECTION('ref_axis',(1.,0.,0.));
#6254=DIRECTION('center_axis',(0.,0.,1.));
#6255=DIRECTION('ref_axis',(1.,0.,0.));
#6256=DIRECTION('',(0.,0.,1.));
#6257=DIRECTION('center_axis',(0.,0.,1.));
#6258=DIRECTION('ref_axis',(1.,0.,0.));
#6259=DIRECTION('center_axis',(0.,0.,1.));
#6260=DIRECTION('ref_axis',(1.,0.,0.));
#6261=DIRECTION('',(0.,0.,1.));
#6262=DIRECTION('center_axis',(0.,0.,1.));
#6263=DIRECTION('ref_axis',(1.,0.,0.));
#6264=DIRECTION('center_axis',(0.,0.,1.));
#6265=DIRECTION('ref_axis',(1.,0.,0.));
#6266=DIRECTION('',(0.,0.,1.));
#6267=DIRECTION('center_axis',(0.,0.,1.));
#6268=DIRECTION('ref_axis',(1.,0.,0.));
#6269=DIRECTION('center_axis',(0.,0.,1.));
#6270=DIRECTION('ref_axis',(1.,0.,0.));
#6271=DIRECTION('center_axis',(0.,0.,1.));
#6272=DIRECTION('ref_axis',(1.,0.,0.));
#6273=DIRECTION('center_axis',(0.,0.,1.));
#6274=DIRECTION('ref_axis',(1.,0.,0.));
#6275=DIRECTION('center_axis',(0.,0.,1.));
#6276=DIRECTION('ref_axis',(1.,0.,0.));
#6277=DIRECTION('',(0.,0.,-1.));
#6278=DIRECTION('center_axis',(0.,0.,1.));
#6279=DIRECTION('ref_axis',(1.,0.,0.));
#6280=DIRECTION('center_axis',(0.,0.,1.));
#6281=DIRECTION('ref_axis',(1.,0.,0.));
#6282=DIRECTION('',(0.,0.,-1.));
#6283=DIRECTION('center_axis',(0.,0.,1.));
#6284=DIRECTION('ref_axis',(1.,0.,0.));
#7593=CARTESIAN_POINT('',(0.,0.,0.));
#7594=CARTESIAN_POINT('Origin',(-0.989949493661167,-0.989949493661166,1.5));
#7595=CARTESIAN_POINT('',(-1.01060488132664,-1.48952266644008,1.5));
#7596=CARTESIAN_POINT('',(-1.48952266644008,-1.01060488132664,1.5));
#7597=CARTESIAN_POINT('Origin',(0.,0.,1.5));
#7598=CARTESIAN_POINT('Origin',(-0.989949493661167,-0.989949493661166,1.5));
#7599=CARTESIAN_POINT('',(-1.26494949366117,-0.989949493661166,1.5));
#7600=CARTESIAN_POINT('Origin',(-0.989949493661167,-0.989949493661166,1.5));
#7601=CARTESIAN_POINT('Origin',(-0.989949493661167,-0.989949493661166,1.5));
#7602=CARTESIAN_POINT('',(-1.01060488132664,-1.48952266644008,2.));
#7603=CARTESIAN_POINT('',(-1.01060488132664,-1.48952266644008,1.5));
#7604=CARTESIAN_POINT('',(-1.48952266644008,-1.01060488132664,2.));
#7605=CARTESIAN_POINT('Origin',(-0.989949493661167,-0.989949493661166,2.));
#7606=CARTESIAN_POINT('',(-1.48952266644008,-1.01060488132664,1.5));
#7607=CARTESIAN_POINT('Origin',(-0.989949493661166,0.989949493661167,1.5));
#7608=CARTESIAN_POINT('',(-1.48952266644008,1.01060488132664,1.5));
#7609=CARTESIAN_POINT('',(-1.01060488132664,1.48952266644008,1.5));
#7610=CARTESIAN_POINT('Origin',(0.,0.,1.5));
#7611=CARTESIAN_POINT('Origin',(-0.989949493661166,0.989949493661167,1.5));
#7612=CARTESIAN_POINT('',(-1.26494949366117,0.989949493661167,1.5));
#7613=CARTESIAN_POINT('Origin',(-0.989949493661166,0.989949493661167,1.5));
#7614=CARTESIAN_POINT('Origin',(-0.989949493661166,0.989949493661167,1.5));
#7615=CARTESIAN_POINT('',(-1.48952266644008,1.01060488132664,2.));
#7616=CARTESIAN_POINT('',(-1.48952266644008,1.01060488132664,1.5));
#7617=CARTESIAN_POINT('',(-1.01060488132664,1.48952266644008,2.));
#7618=CARTESIAN_POINT('Origin',(-0.989949493661166,0.989949493661167,2.));
#7619=CARTESIAN_POINT('',(-1.01060488132664,1.48952266644008,1.5));
#7620=CARTESIAN_POINT('Origin',(0.989949493661167,0.989949493661166,1.5));
#7621=CARTESIAN_POINT('',(1.01060488132664,1.48952266644008,1.5));
#7622=CARTESIAN_POINT('',(1.48952266644008,1.01060488132664,1.5));
#7623=CARTESIAN_POINT('Origin',(0.,0.,1.5));
#7624=CARTESIAN_POINT('Origin',(0.989949493661167,0.989949493661166,1.5));
#7625=CARTESIAN_POINT('',(0.714949493661166,0.989949493661166,1.5));
#7626=CARTESIAN_POINT('Origin',(0.989949493661167,0.989949493661166,1.5));
#7627=CARTESIAN_POINT('Origin',(0.989949493661167,0.989949493661166,1.5));
#7628=CARTESIAN_POINT('',(1.01060488132664,1.48952266644008,2.));
#7629=CARTESIAN_POINT('',(1.01060488132664,1.48952266644008,1.5));
#7630=CARTESIAN_POINT('',(1.48952266644008,1.01060488132664,2.));
#7631=CARTESIAN_POINT('Origin',(0.989949493661167,0.989949493661166,2.));
#7632=CARTESIAN_POINT('',(1.48952266644008,1.01060488132664,1.5));
#7633=CARTESIAN_POINT('Origin',(0.989949493661166,-0.989949493661167,1.5));
#7634=CARTESIAN_POINT('',(1.48952266644008,-1.01060488132664,1.5));
#7635=CARTESIAN_POINT('',(1.01060488132664,-1.48952266644008,1.5));
#7636=CARTESIAN_POINT('Origin',(0.,0.,1.5));
#7637=CARTESIAN_POINT('Origin',(0.989949493661166,-0.989949493661167,1.5));
#7638=CARTESIAN_POINT('',(0.714949493661166,-0.989949493661167,1.5));
#7639=CARTESIAN_POINT('Origin',(0.989949493661166,-0.989949493661167,1.5));
#7640=CARTESIAN_POINT('Origin',(0.989949493661166,-0.989949493661167,1.5));
#7641=CARTESIAN_POINT('',(1.48952266644008,-1.01060488132664,2.));
#7642=CARTESIAN_POINT('',(1.48952266644008,-1.01060488132664,1.5));
#7643=CARTESIAN_POINT('',(1.01060488132664,-1.48952266644008,2.));
#7644=CARTESIAN_POINT('Origin',(0.989949493661166,-0.989949493661167,2.));
#7645=CARTESIAN_POINT('',(1.01060488132664,-1.48952266644008,1.5));
#7646=CARTESIAN_POINT('Origin',(0.,0.,2.));
#7647=CARTESIAN_POINT('Origin',(0.,0.,2.));
#7648=CARTESIAN_POINT('Origin',(0.,0.,2.));
#7649=CARTESIAN_POINT('Origin',(0.,0.,2.));
#7650=CARTESIAN_POINT('',(-1.8,-2.20436423846524E-16,2.));
#7651=CARTESIAN_POINT('Origin',(0.,0.,2.));
#7652=CARTESIAN_POINT('Origin',(0.,0.,2.));
#7653=CARTESIAN_POINT('',(-0.5,-6.12323399573677E-17,2.));
#7654=CARTESIAN_POINT('Origin',(0.,0.,2.));
#7655=CARTESIAN_POINT('Origin',(0.,0.,1.));
#7656=CARTESIAN_POINT('',(-1.8,-2.20436423846524E-16,1.));
#7657=CARTESIAN_POINT('',(-1.8,-2.20436423846524E-16,1.));
#7658=CARTESIAN_POINT('Origin',(0.,0.,1.));
#7659=CARTESIAN_POINT('Origin',(-2.31008116418808,-5.,9.02921777339027));
#7660=CARTESIAN_POINT('',(-2.61008116418808,-1.4,9.02921777339027));
#7661=CARTESIAN_POINT('Origin',(-2.31008116418808,-1.4,9.02921777339027));
#7662=CARTESIAN_POINT('',(-2.61008116418808,-5.,9.02921777339027));
#7663=CARTESIAN_POINT('',(-2.61008116418808,-5.,9.02921777339027));
#7664=CARTESIAN_POINT('Origin',(-2.31008116418808,-5.,9.02921777339027));
#7665=CARTESIAN_POINT('Origin',(-2.31008116418808,-1.4,9.02921777339027));
#7666=CARTESIAN_POINT('Origin',(-1.5,-5.,13.5));
#7667=CARTESIAN_POINT('',(-1.,-5.,18.5));
#7668=CARTESIAN_POINT('',(-1.,-5.,19.));
#7669=CARTESIAN_POINT('',(-1.,-5.,16.));
#7670=CARTESIAN_POINT('',(0.,-5.,18.5));
#7671=CARTESIAN_POINT('',(-0.75,-5.,18.5));
#7672=CARTESIAN_POINT('',(0.,-5.,8.));
#7673=CARTESIAN_POINT('',(0.,-5.,8.));
#7674=CARTESIAN_POINT('',(-3.,-5.,8.));
#7675=CARTESIAN_POINT('',(-3.,-5.,8.));
#7676=CARTESIAN_POINT('',(-3.,-5.,19.));
#7677=CARTESIAN_POINT('',(-3.,-5.,19.));
#7678=CARTESIAN_POINT('',(0.,-5.,19.));
#7679=CARTESIAN_POINT('Origin',(0.,-5.5,19.));
#7680=CARTESIAN_POINT('',(0.,-5.5,18.5));
#7681=CARTESIAN_POINT('',(0.,-4.125,18.5));
#7682=CARTESIAN_POINT('',(0.,-5.5,8.));
#7683=CARTESIAN_POINT('',(0.,-5.5,8.));
#7684=CARTESIAN_POINT('',(0.,-5.5,8.));
#7685=CARTESIAN_POINT('Origin',(-3.,-5.5,8.));
#7686=CARTESIAN_POINT('',(-3.,-5.5,19.));
#7687=CARTESIAN_POINT('',(-3.,-5.5,8.));
#7688=CARTESIAN_POINT('',(-3.,-5.5,19.));
#7689=CARTESIAN_POINT('',(-3.,-5.5,19.));
#7690=CARTESIAN_POINT('',(-3.,-5.5,8.));
#7691=CARTESIAN_POINT('Origin',(0.,-5.5,8.));
#7692=CARTESIAN_POINT('',(-3.,-5.5,8.));
#7693=CARTESIAN_POINT('Origin',(-1.,0.,18.5));
#7694=CARTESIAN_POINT('',(-1.,0.,19.));
#7695=CARTESIAN_POINT('',(-1.,0.,19.));
#7696=CARTESIAN_POINT('',(-1.,0.,18.5));
#7697=CARTESIAN_POINT('',(-1.,0.,18.5));
#7698=CARTESIAN_POINT('',(-1.,0.,18.5));
#7699=CARTESIAN_POINT('Origin',(0.,0.,19.));
#7700=CARTESIAN_POINT('',(1.,-5.5,19.));
#7701=CARTESIAN_POINT('',(0.,-5.5,19.));
#7702=CARTESIAN_POINT('',(1.,0.,19.));
#7703=CARTESIAN_POINT('',(1.,-5.5,19.));
#7704=CARTESIAN_POINT('',(0.5,0.,19.));
#7705=CARTESIAN_POINT('',(1.,0.,19.));
#7706=CARTESIAN_POINT('',(-0.5,-6.12323399573677E-17,19.));
#7707=CARTESIAN_POINT('Origin',(0.,0.,19.));
#7708=CARTESIAN_POINT('',(1.,0.,19.));
#7709=CARTESIAN_POINT('Origin',(1.,0.,18.5));
#7710=CARTESIAN_POINT('',(-0.5,0.,18.5));
#7711=CARTESIAN_POINT('',(-0.5,0.,12.));
#7712=CARTESIAN_POINT('',(1.,0.,18.5));
#7713=CARTESIAN_POINT('Origin',(1.,0.,18.5));
#7714=CARTESIAN_POINT('',(0.5,0.,18.5));
#7715=CARTESIAN_POINT('',(0.5,0.,12.));
#7716=CARTESIAN_POINT('',(1.,0.,18.5));
#7717=CARTESIAN_POINT('',(1.,0.,18.5));
#7718=CARTESIAN_POINT('',(1.,0.,18.5));
#7719=CARTESIAN_POINT('Origin',(1.,-5.5,18.5));
#7720=CARTESIAN_POINT('',(1.,-5.5,18.5));
#7721=CARTESIAN_POINT('',(1.,-5.5,18.5));
#7722=CARTESIAN_POINT('',(1.,-5.5,18.5));
#7723=CARTESIAN_POINT('Origin',(-1.,-5.5,18.5));
#7724=CARTESIAN_POINT('',(-1.,-5.5,18.5));
#7725=CARTESIAN_POINT('Origin',(0.,-2.75,18.5));
#7726=CARTESIAN_POINT('Origin',(0.,0.,18.5));
#7727=CARTESIAN_POINT('Origin',(0.,0.,12.));
#7728=CARTESIAN_POINT('',(-0.5,-6.12323399573677E-17,12.));
#7729=CARTESIAN_POINT('',(-0.5,-6.12323399573677E-17,12.));
#7730=CARTESIAN_POINT('Origin',(0.,0.,12.));
#7731=CARTESIAN_POINT('',(0.,-0.5,12.2));
#7732=CARTESIAN_POINT('',(0.,-0.5,12.7));
#7733=CARTESIAN_POINT('',(0.,-0.5,12.));
#7734=CARTESIAN_POINT('',(0.3,-0.4,12.7));
#7735=CARTESIAN_POINT('Origin',(0.,0.,12.7));
#7736=CARTESIAN_POINT('',(0.3,-0.4,12.2));
#7737=CARTESIAN_POINT('',(0.3,-0.4,12.));
#7738=CARTESIAN_POINT('Origin',(0.,0.,12.2));
#7739=CARTESIAN_POINT('',(0.,0.5,12.7));
#7740=CARTESIAN_POINT('',(0.,0.5,12.2));
#7741=CARTESIAN_POINT('',(0.,0.5,12.));
#7742=CARTESIAN_POINT('',(0.3,0.4,12.2));
#7743=CARTESIAN_POINT('Origin',(0.,0.,12.2));
#7744=CARTESIAN_POINT('',(0.3,0.4,12.7));
#7745=CARTESIAN_POINT('',(0.3,0.4,12.));
#7746=CARTESIAN_POINT('Origin',(0.,0.,12.7));
#7747=CARTESIAN_POINT('Origin',(2.,0.6,10.5));
#7748=CARTESIAN_POINT('',(1.695,0.7,10.5));
#7749=CARTESIAN_POINT('Origin',(2.,0.7,10.5));
#7750=CARTESIAN_POINT('',(1.695,1.4,10.5));
#7751=CARTESIAN_POINT('',(1.695,0.6,10.5));
#7752=CARTESIAN_POINT('Origin',(2.,1.4,10.5));
#7753=CARTESIAN_POINT('Origin',(1.,0.7,12.5));
#7754=CARTESIAN_POINT('',(3.,0.7,12.5));
#7755=CARTESIAN_POINT('',(3.,1.4,12.5));
#7756=CARTESIAN_POINT('',(3.,0.55,12.5));
#7757=CARTESIAN_POINT('',(3.5,0.7,12.5));
#7758=CARTESIAN_POINT('',(3.5,0.7,12.5));
#7759=CARTESIAN_POINT('',(3.5,1.4,12.5));
#7760=CARTESIAN_POINT('',(3.5,0.7,12.5));
#7761=CARTESIAN_POINT('',(3.5,1.4,12.5));
#7762=CARTESIAN_POINT('Origin',(1.,0.7,9.5));
#7763=CARTESIAN_POINT('',(1.,1.4,12.2));
#7764=CARTESIAN_POINT('',(1.,0.7,12.2));
#7765=CARTESIAN_POINT('',(1.,0.55,12.2));
#7766=CARTESIAN_POINT('',(1.,1.4,9.5));
#7767=CARTESIAN_POINT('',(1.,1.4,12.5));
#7768=CARTESIAN_POINT('',(1.,0.7,9.5));
#7769=CARTESIAN_POINT('',(1.,0.7,9.5));
#7770=CARTESIAN_POINT('',(1.,0.7,12.5));
#7771=CARTESIAN_POINT('Origin',(3.5,0.7,9.5));
#7772=CARTESIAN_POINT('',(3.5,0.7,9.5));
#7773=CARTESIAN_POINT('',(1.,0.7,9.5));
#7774=CARTESIAN_POINT('',(3.5,1.4,9.5));
#7775=CARTESIAN_POINT('',(1.,1.4,9.5));
#7776=CARTESIAN_POINT('',(3.5,0.7,9.5));
#7777=CARTESIAN_POINT('Origin',(3.5,0.7,12.5));
#7778=CARTESIAN_POINT('',(3.5,0.7,9.5));
#7779=CARTESIAN_POINT('',(3.5,1.4,9.5));
#7780=CARTESIAN_POINT('Origin',(2.25,0.7,11.));
#7781=CARTESIAN_POINT('',(3.,0.7,12.2));
#7782=CARTESIAN_POINT('',(2.625,0.7,12.2));
#7783=CARTESIAN_POINT('',(3.,0.7,11.85));
#7784=CARTESIAN_POINT('Origin',(3.,0.4,12.2));
#7785=CARTESIAN_POINT('',(3.,0.4,12.2));
#7786=CARTESIAN_POINT('',(3.,0.4,12.2));
#7787=CARTESIAN_POINT('',(0.,0.4,12.2));
#7788=CARTESIAN_POINT('',(0.,1.4,12.2));
#7789=CARTESIAN_POINT('',(0.,0.4,12.2));
#7790=CARTESIAN_POINT('',(0.,1.4,12.2));
#7791=CARTESIAN_POINT('Origin',(3.,0.4,12.7));
#7792=CARTESIAN_POINT('',(3.,1.4,12.7));
#7793=CARTESIAN_POINT('',(3.,1.4,12.2));
#7794=CARTESIAN_POINT('',(3.,0.4,12.7));
#7795=CARTESIAN_POINT('',(3.,0.4,12.7));
#7796=CARTESIAN_POINT('',(3.,0.4,12.2));
#7797=CARTESIAN_POINT('Origin',(0.,0.4,12.2));
#7798=CARTESIAN_POINT('',(0.,1.4,12.7));
#7799=CARTESIAN_POINT('',(0.,0.4,12.7));
#7800=CARTESIAN_POINT('',(0.,1.4,12.7));
#7801=CARTESIAN_POINT('Origin',(0.,0.4,12.7));
#7802=CARTESIAN_POINT('',(3.,0.4,12.7));
#7803=CARTESIAN_POINT('',(3.,1.4,12.7));
#7804=CARTESIAN_POINT('Origin',(1.5,1.4,12.45));
#7805=CARTESIAN_POINT('Origin',(1.5,0.4,12.45));
#7806=CARTESIAN_POINT('Origin',(2.,-1.5,10.5));
#7807=CARTESIAN_POINT('',(1.695,-1.4,10.5));
#7808=CARTESIAN_POINT('Origin',(2.,-1.4,10.5));
#7809=CARTESIAN_POINT('',(1.695,-0.7,10.5));
#7810=CARTESIAN_POINT('',(1.695,-1.5,10.5));
#7811=CARTESIAN_POINT('Origin',(2.,-0.7,10.5));
#7812=CARTESIAN_POINT('Origin',(2.25,-0.7,11.));
#7813=CARTESIAN_POINT('',(3.,-0.7,12.2));
#7814=CARTESIAN_POINT('',(1.,-0.7,12.2));
#7815=CARTESIAN_POINT('',(2.625,-0.7,12.2));
#7816=CARTESIAN_POINT('',(3.,-0.7,12.5));
#7817=CARTESIAN_POINT('',(3.,-0.7,11.85));
#7818=CARTESIAN_POINT('',(3.5,-0.7,12.5));
#7819=CARTESIAN_POINT('',(3.5,-0.7,12.5));
#7820=CARTESIAN_POINT('',(3.5,-0.7,9.5));
#7821=CARTESIAN_POINT('',(3.5,-0.7,9.5));
#7822=CARTESIAN_POINT('',(1.,-0.7,9.5));
#7823=CARTESIAN_POINT('',(1.,-0.7,9.5));
#7824=CARTESIAN_POINT('',(1.,-0.7,12.5));
#7825=CARTESIAN_POINT('Origin',(1.,-1.4,12.5));
#7826=CARTESIAN_POINT('',(3.,-1.4,12.5));
#7827=CARTESIAN_POINT('',(3.,-1.4,12.5));
#7828=CARTESIAN_POINT('',(3.5,-1.4,12.5));
#7829=CARTESIAN_POINT('',(3.5,-1.4,12.5));
#7830=CARTESIAN_POINT('',(3.5,-1.4,12.5));
#7831=CARTESIAN_POINT('Origin',(1.,-1.4,9.5));
#7832=CARTESIAN_POINT('',(1.,-1.4,12.2));
#7833=CARTESIAN_POINT('',(1.,-1.4,12.2));
#7834=CARTESIAN_POINT('',(1.,-1.4,9.5));
#7835=CARTESIAN_POINT('',(1.,-1.4,9.5));
#7836=CARTESIAN_POINT('',(1.,-1.4,12.5));
#7837=CARTESIAN_POINT('Origin',(3.5,-1.4,9.5));
#7838=CARTESIAN_POINT('',(3.5,-1.4,9.5));
#7839=CARTESIAN_POINT('',(1.,-1.4,9.5));
#7840=CARTESIAN_POINT('',(3.5,-1.4,9.5));
#7841=CARTESIAN_POINT('Origin',(3.5,-1.4,12.5));
#7842=CARTESIAN_POINT('',(3.5,-1.4,9.5));
#7843=CARTESIAN_POINT('Origin',(1.5,-1.4,12.45));
#7844=CARTESIAN_POINT('',(3.,-1.4,12.7));
#7845=CARTESIAN_POINT('',(3.,-1.4,12.2));
#7846=CARTESIAN_POINT('',(0.,-1.4,12.7));
#7847=CARTESIAN_POINT('',(3.,-1.4,12.7));
#7848=CARTESIAN_POINT('',(0.,-1.4,12.2));
#7849=CARTESIAN_POINT('',(0.,-1.4,12.7));
#7850=CARTESIAN_POINT('',(0.,-1.4,12.2));
#7851=CARTESIAN_POINT('Origin',(0.,-1.4,12.7));
#7852=CARTESIAN_POINT('',(0.,-1.4,12.7));
#7853=CARTESIAN_POINT('',(3.,-0.4,12.7));
#7854=CARTESIAN_POINT('',(3.,-1.4,12.7));
#7855=CARTESIAN_POINT('',(3.,-0.4,12.7));
#7856=CARTESIAN_POINT('Origin',(0.,-1.4,12.2));
#7857=CARTESIAN_POINT('',(0.,-1.4,12.2));
#7858=CARTESIAN_POINT('Origin',(3.,-1.4,12.2));
#7859=CARTESIAN_POINT('',(3.,-0.4,12.2));
#7860=CARTESIAN_POINT('',(0.,-0.4,12.2));
#7861=CARTESIAN_POINT('',(3.,-1.4,12.2));
#7862=CARTESIAN_POINT('Origin',(3.,-1.4,12.7));
#7863=CARTESIAN_POINT('',(3.,-0.4,12.2));
#7864=CARTESIAN_POINT('Origin',(1.5,-0.4,12.45));
#7865=CARTESIAN_POINT('Origin',(-0.989949493661167,-0.989949493661166,0.9));
#7866=CARTESIAN_POINT('',(-1.26494949366117,-0.989949493661166,1.));
#7867=CARTESIAN_POINT('Origin',(-0.989949493661167,-0.989949493661166,1.));
#7868=CARTESIAN_POINT('',(-1.26494949366117,-0.989949493661166,0.9));
#7869=CARTESIAN_POINT('Origin',(-0.989949493661166,0.989949493661167,0.9));
#7870=CARTESIAN_POINT('',(-1.26494949366117,0.989949493661167,1.));
#7871=CARTESIAN_POINT('Origin',(-0.989949493661166,0.989949493661167,1.));
#7872=CARTESIAN_POINT('',(-1.26494949366117,0.989949493661167,0.9));
#7873=CARTESIAN_POINT('Origin',(0.989949493661167,0.989949493661166,0.9));
#7874=CARTESIAN_POINT('',(0.714949493661166,0.989949493661166,1.));
#7875=CARTESIAN_POINT('Origin',(0.989949493661167,0.989949493661166,1.));
#7876=CARTESIAN_POINT('',(0.714949493661166,0.989949493661166,0.9));
#7877=CARTESIAN_POINT('Origin',(0.989949493661166,-0.989949493661167,0.9));
#7878=CARTESIAN_POINT('',(0.714949493661166,-0.989949493661167,1.));
#7879=CARTESIAN_POINT('Origin',(0.989949493661166,-0.989949493661167,1.));
#7880=CARTESIAN_POINT('',(0.714949493661166,-0.989949493661167,0.9));
#7881=CARTESIAN_POINT('Origin',(0.,0.,11.));
#7882=CARTESIAN_POINT('',(-0.7,-8.57252759403147E-17,11.));
#7883=CARTESIAN_POINT('Origin',(0.,0.,11.));
#7884=CARTESIAN_POINT('',(-0.5,-6.12323399573677E-17,11.));
#7885=CARTESIAN_POINT('Origin',(0.,0.,11.));
#7886=CARTESIAN_POINT('Origin',(0.,0.,11.));
#7887=CARTESIAN_POINT('',(-0.7,-8.57252759403147E-17,12.));
#7888=CARTESIAN_POINT('Origin',(0.,0.,12.));
#7889=CARTESIAN_POINT('',(-0.7,-8.57252759403147E-17,11.));
#7890=CARTESIAN_POINT('Origin',(0.,0.,12.));
#7891=CARTESIAN_POINT('Origin',(0.,0.,2.));
#7892=CARTESIAN_POINT('',(-0.5,-6.12323399573677E-17,2.));
#7893=CARTESIAN_POINT('Origin',(0.,0.,1.));
#10569=UNCERTAINTY_MEASURE_WITH_UNIT(LENGTH_MEASURE(0.001),#10628,
'DISTANCE_ACCURACY_VALUE',
'Maximum model space distance between geometric entities at asserted c
onnectivities');
#10595=UNCERTAINTY_MEASURE_WITH_UNIT(LENGTH_MEASURE(0.001),#10628,
'DISTANCE_ACCURACY_VALUE',
'Maximum model space distance between geometric entities at asserted c
onnectivities');
#10601=(
GEOMETRIC_REPRESENTATION_CONTEXT(3)
GLOBAL_UNCERTAINTY_ASSIGNED_CONTEXT((#10569))
GLOBAL_UNIT_ASSIGNED_CONTEXT((#10628,#10630,#10631))
REPRESENTATION_CONTEXT('','3D')
);
#10627=(
GEOMETRIC_REPRESENTATION_CONTEXT(3)
GLOBAL_UNCERTAINTY_ASSIGNED_CONTEXT((#10595))
GLOBAL_UNIT_ASSIGNED_CONTEXT((#10628,#10630,#10631))
REPRESENTATION_CONTEXT('','3D')
);
#10628=(
LENGTH_UNIT()
NAMED_UNIT(*)
SI_UNIT(.CENTI.,.METRE.)
);
#10630=(
NAMED_UNIT(*)
PLANE_ANGLE_UNIT()
SI_UNIT($,.RADIAN.)
);
#10631=(
NAMED_UNIT(*)
SI_UNIT($,.STERADIAN.)
SOLID_ANGLE_UNIT()
);
#10637=SHAPE_DEFINITION_REPRESENTATION(#10668,#10742);
#10668=PRODUCT_DEFINITION_SHAPE('',$,#10774);
#10742=SHAPE_REPRESENTATION('',(#5258),#10601);
#10768=PRODUCT_DEFINITION_CONTEXT('part definition',#10863,'design');
#10774=PRODUCT_DEFINITION('Post and cam fork','Post and cam fork',#10805,
#10768);
#10805=PRODUCT_DEFINITION_FORMATION('',$,#10870);
#10863=APPLICATION_CONTEXT(
'Core Data for Automotive Mechanical Design Process');
#10864=PRODUCT_CONTEXT('part definition',#10863,'mechanical');
#10870=PRODUCT('Post and cam fork','Post and cam fork',
'Post and cam fork',(#10864));
#10952=COLOUR_RGB('Sky Blue',0.24,0.69,0.87);
#10953=FILL_AREA_STYLE_COLOUR('',#10952);
#10954=FILL_AREA_STYLE('',(#10953));
#10955=SURFACE_STYLE_FILL_AREA(#10954);
#10956=SURFACE_SIDE_STYLE('',(#10955));
#10957=SURFACE_STYLE_USAGE(.BOTH.,#10956);
#10958=PRESENTATION_STYLE_ASSIGNMENT((#10957));
ENDSEC;
END-ISO-10303-21;
